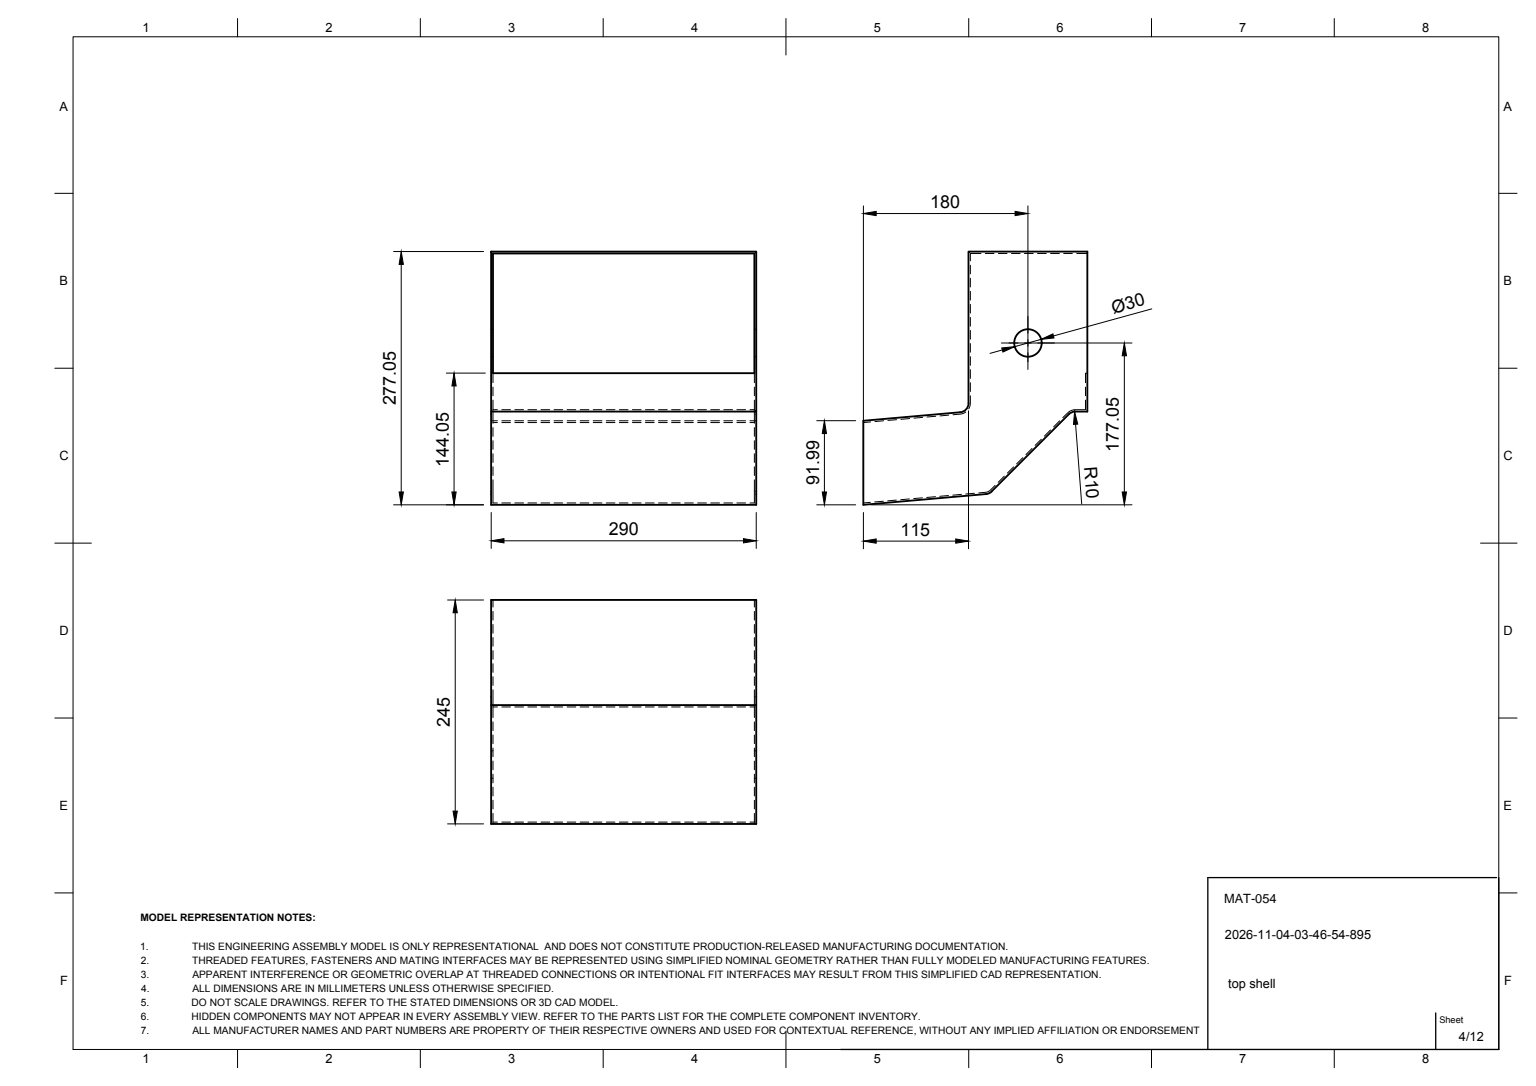
ISO-10303-21;
HEADER;
FILE_DESCRIPTION (('STEP AP214'),
    '1' );
FILE_NAME ('top shell.step',
    '2026-10-21T17:50:41',
    ( '' ),
    ( '' ),
    'SwSTEP 2.0',
    'SolidWorks 2026',
    '' );
FILE_SCHEMA (( 'AUTOMOTIVE_DESIGN' ));
ENDSEC;

DATA;
#13=ORIENTED_EDGE ( 'NONE', *, *, #11369, .F. ) ;
#14=DIRECTION ( 'NONE',  ( 0.000000000000000000, 0.000000000000000000, -1.000000000000000000 ) ) ;
#111=DIRECTION ( 'NONE',  ( -1.000000000000000000, -0.000000000000000000, 0.000000000000000000 ) ) ;
#224=CARTESIAN_POINT ( 'NONE',  ( 143.0000000000000568, -90.29102463692673552, -73.95413108702813076 ) ) ;
#230=LINE ( 'NONE', #27103, #6038 ) ;
#238=DIRECTION ( 'NONE',  ( 0.000000000000000000, 0.000000000000000000, 1.000000000000000000 ) ) ;
#332=VECTOR ( 'NONE', #22185, 999.9999999999998863 ) ;
#381=EDGE_CURVE ( 'NONE', #23842, #27991, #33323, .T. ) ;
#384=CARTESIAN_POINT ( 'NONE',  ( 145.0000000000000568, -87.50000000000000000, 65.00000000000000000 ) ) ;
#404=VERTEX_POINT ( 'NONE', #32954 ) ;
#417=EDGE_CURVE ( 'NONE', #26117, #20828, #25120, .T. ) ;
#450=ORIENTED_EDGE ( 'NONE', *, *, #30527, .F. ) ;
#467=CARTESIAN_POINT ( 'NONE',  ( -145.0000000000000568, -87.50000000000000000, 65.00000000000000000 ) ) ;
#474=VERTEX_POINT ( 'NONE', #30482 ) ;
#477=DIRECTION ( 'NONE',  ( 0.000000000000000000, 0.000000000000000000, 1.000000000000000000 ) ) ;
#478=CARTESIAN_POINT ( 'NONE',  ( 145.0000000000000568, -90.29102463692674974, -73.95413108702814498 ) ) ;
#501=VERTEX_POINT ( 'NONE', #14993 ) ;
#508=EDGE_CURVE ( 'NONE', #6161, #17092, #29208, .T. ) ;
#579=DIRECTION ( 'NONE',  ( -1.000000000000000000, -0.000000000000000000, -0.000000000000000000 ) ) ;
#608=AXIS2_PLACEMENT_3D ( 'NONE', #24658, #22008, #32850 ) ;
#649=FACE_OUTER_BOUND ( 'NONE', #15663, .T. ) ;
#660=VECTOR ( 'NONE', #33698, 1000.000000000000000 ) ;
#691=DIRECTION ( 'NONE',  ( -1.000000000000000000, -0.000000000000000000, -0.000000000000000000 ) ) ;
#694=ORIENTED_EDGE ( 'NONE', *, *, #22904, .F. ) ;
#716=LINE ( 'NONE', #33098, #30982 ) ;
#751=CARTESIAN_POINT ( 'NONE',  ( 143.0000000000000568, -167.8552739801376390, -46.75049602362128809 ) ) ;
#757=DIRECTION ( 'NONE',  ( -1.000000000000000000, -0.000000000000000000, -0.000000000000000000 ) ) ;
#923=ORIENTED_EDGE ( 'NONE', *, *, #10157, .T. ) ;
#932=DIRECTION ( 'NONE',  ( 0.000000000000000000, 0.000000000000000000, -1.000000000000000000 ) ) ;
#975=LINE ( 'NONE', #1321, #16054 ) ;
#984=VERTEX_POINT ( 'NONE', #15788 ) ;
#990=AXIS2_PLACEMENT_3D ( 'NONE', #24668, #10640, #10812 ) ;
#1006=LINE ( 'NONE', #478, #28288 ) ;
#1010=CARTESIAN_POINT ( 'NONE',  ( 145.0000000000000568, -99.56883598056833762, -180.0000000000000000 ) ) ;
#1039=CARTESIAN_POINT ( 'NONE',  ( 187.4264068711928530, -12.50000000000001066, 15.00000000000001243 ) ) ;
#1054=VERTEX_POINT ( 'NONE', #18119 ) ;
#1114=MECHANICAL_DESIGN_GEOMETRIC_PRESENTATION_REPRESENTATION('',(#28951),#30096);
#1116=SHAPE_REPRESENTATION_RELATIONSHIP ( 'NONE' , 'NONE' ,  #34141, #15654 ) ;
#1119=VECTOR ( 'NONE', #9651, 1000.000000000000000 ) ;
#1129=VECTOR ( 'NONE', #24012, 1000.000000000000000 ) ;
#1146=ORIENTED_EDGE ( 'NONE', *, *, #20627, .F. ) ;
#1160=ORIENTED_EDGE ( 'NONE', *, *, #15687, .T. ) ;
#1162=ADVANCED_FACE ( 'NONE', ( #33539, #17379 ), #31058, .F. ) ;
#1184=DIRECTION ( 'NONE',  ( 0.000000000000000000, 0.000000000000000000, 1.000000000000000000 ) ) ;
#1244=ORIENTED_EDGE ( 'NONE', *, *, #5386, .F. ) ;
#1280=DIRECTION ( 'NONE',  ( 0.000000000000000000, 1.000000000000000000, 0.000000000000000000 ) ) ;
#1321=CARTESIAN_POINT ( 'NONE',  ( 145.0000000000000568, -97.56119630548165844, -180.0000000000000000 ) ) ;
#1392=ORIENTED_EDGE ( 'NONE', *, *, #20061, .F. ) ;
#1406=ORIENTED_EDGE ( 'NONE', *, *, #28646, .F. ) ;
#1446=ORIENTED_EDGE ( 'NONE', *, *, #32975, .T. ) ;
#1462=EDGE_CURVE ( 'NONE', #30062, #4232, #230, .T. ) ;
#1493=DIRECTION ( 'NONE',  ( 0.000000000000000000, 0.000000000000000000, 1.000000000000000000 ) ) ;
#1495=EDGE_CURVE ( 'NONE', #13296, #6161, #27458, .T. ) ;
#1497=FACE_OUTER_BOUND ( 'NONE', #34932, .T. ) ;
#1609=ORIENTED_EDGE ( 'NONE', *, *, #17986, .F. ) ;
#1662=CARTESIAN_POINT ( 'NONE',  ( 145.0000000000000568, -167.8552739801376390, -46.75049602362128809 ) ) ;
#1668=CARTESIAN_POINT ( 'NONE',  ( 145.0000000000000568, -97.49999999999998579, 51.88904920397793319 ) ) ;
#1722=VERTEX_POINT ( 'NONE', #2207 ) ;
#1762=ORIENTED_EDGE ( 'NONE', *, *, #9120, .F. ) ;
#1828=VECTOR ( 'NONE', #34629, 1000.000000000000000 ) ;
#1964=ORIENTED_EDGE ( 'NONE', *, *, #8386, .F. ) ;
#1974=DIRECTION ( 'NONE',  ( -1.000000000000000000, -0.000000000000000000, -0.000000000000000000 ) ) ;
#2049=UNCERTAINTY_MEASURE_WITH_UNIT (LENGTH_MEASURE( 1.000000000000000082E-05 ), #3564, 'distance_accuracy_value', 'NONE');
#2074=EDGE_CURVE ( 'NONE', #21429, #4511, #10494, .T. ) ;
#2104=ORIENTED_EDGE ( 'NONE', *, *, #27915, .T. ) ;
#2107=EDGE_LOOP ( 'NONE', ( #4532, #34179, #24526, #34171 ) ) ;
#2147=DIRECTION ( 'NONE',  ( -0.000000000000000000, 1.000000000000000000, 0.000000000000000000 ) ) ;
#2200=DIRECTION ( 'NONE',  ( 0.000000000000000000, 0.000000000000000000, 1.000000000000000000 ) ) ;
#2207=CARTESIAN_POINT ( 'NONE',  ( 143.0000000000000568, -175.8248315648716016, -46.05325008164005851 ) ) ;
#2212=DIRECTION ( 'NONE',  ( 0.000000000000000000, -0.000000000000000000, -1.000000000000000000 ) ) ;
#2216=LINE ( 'NONE', #23916, #17432 ) ;
#2264=ORIENTED_EDGE ( 'NONE', *, *, #32975, .F. ) ;
#2305=FACE_OUTER_BOUND ( 'NONE', #6168, .T. ) ;
#2345=FACE_OUTER_BOUND ( 'NONE', #21509, .T. ) ;
#2382=ORIENTED_EDGE ( 'NONE', *, *, #15611, .F. ) ;
#2386=EDGE_CURVE ( 'NONE', #32063, #28687, #25581, .T. ) ;
#2423=DIRECTION ( 'NONE',  ( 1.000000000000000000, 0.000000000000000000, 0.000000000000000000 ) ) ;
#2439=VERTEX_POINT ( 'NONE', #30935 ) ;
#2538=VECTOR ( 'NONE', #8049, 999.9999999999998863 ) ;
#2546=DIRECTION ( 'NONE',  ( -1.000000000000000000, -0.000000000000000000, -0.000000000000000000 ) ) ;
#2625=DIRECTION ( 'NONE',  ( 0.000000000000000000, 0.000000000000000000, -1.000000000000000000 ) ) ;
#2626=ORIENTED_EDGE ( 'NONE', *, *, #4967, .F. ) ;
#2671=CARTESIAN_POINT ( 'NONE',  ( 145.0000000000000568, -87.50000000000000000, 65.00000000000000000 ) ) ;
#2701=DIRECTION ( 'NONE',  ( 0.000000000000000000, 0.08715574274765885976, 0.9961946980917454342 ) ) ;
#2717=CARTESIAN_POINT ( 'NONE',  ( 145.0000000000000568, -177.8172209610550851, -45.87893859614474223 ) ) ;
#2748=DIRECTION ( 'NONE',  ( -1.000000000000000000, -0.000000000000000000, -0.000000000000000000 ) ) ;
#2766=ADVANCED_FACE ( 'NONE', ( #12390 ), #33735, .T. ) ;
#2827=ORIENTED_EDGE ( 'NONE', *, *, #11782, .F. ) ;
#2895=EDGE_LOOP ( 'NONE', ( #29008, #11211, #28715, #34782, #8518, #32872, #13532, #19129, #17560, #923, #20347, #17292, #33269 ) ) ;
#2907=ADVANCED_FACE ( 'NONE', ( #26592 ), #20740, .T. ) ;
#2992=ORIENTED_EDGE ( 'NONE', *, *, #10272, .F. ) ;
#3001=VERTEX_POINT ( 'NONE', #32627 ) ;
#3070=VECTOR ( 'NONE', #20545, 999.9999999999998863 ) ;
#3081=EDGE_CURVE ( 'NONE', #20828, #6161, #16397, .T. ) ;
#3110=AXIS2_PLACEMENT_3D ( 'NONE', #24223, #10182, #23528 ) ;
#3175=VERTEX_POINT ( 'NONE', #17168 ) ;
#3206=ORIENTED_EDGE ( 'NONE', *, *, #4973, .T. ) ;
#3237=FACE_OUTER_BOUND ( 'NONE', #2895, .T. ) ;
#3262=DIRECTION ( 'NONE',  ( 0.000000000000000000, 0.000000000000000000, -1.000000000000000000 ) ) ;
#3299=DIRECTION ( 'NONE',  ( 0.000000000000000000, 0.000000000000000000, -1.000000000000000000 ) ) ;
#3328=LINE ( 'NONE', #22377, #8717 ) ;
#3329=EDGE_LOOP ( 'NONE', ( #28799, #16866, #1609, #5261 ) ) ;
#3333=ORIENTED_EDGE ( 'NONE', *, *, #18846, .F. ) ;
#3359=EDGE_CURVE ( 'NONE', #26117, #13296, #26604, .T. ) ;
#3458=ORIENTED_EDGE ( 'NONE', *, *, #1462, .F. ) ;
#3475=AXIS2_PLACEMENT_3D ( 'NONE', #25994, #12657, #33480 ) ;
#3486=DIRECTION ( 'NONE',  ( 0.000000000000000000, 0.000000000000000000, -1.000000000000000000 ) ) ;
#3544=CARTESIAN_POINT ( 'NONE',  ( 143.0000000000000568, -78.33668825982573480, -63.00000000000000000 ) ) ;
#3564=( LENGTH_UNIT ( ) NAMED_UNIT ( * ) SI_UNIT ( .MILLI., .METRE. ) );
#3617=DIRECTION ( 'NONE',  ( 0.000000000000000000, -0.7071067811865489050, -0.7071067811865462405 ) ) ;
#3629=CARTESIAN_POINT ( 'NONE',  ( -143.0000000000000568, -12.50000000000001066, 15.00000000000001243 ) ) ;
#3804=LINE ( 'NONE', #31730, #14481 ) ;
#3827=ORIENTED_EDGE ( 'NONE', *, *, #20467, .T. ) ;
#3841=ORIENTED_EDGE ( 'NONE', *, *, #34221, .F. ) ;
#3928=CARTESIAN_POINT ( 'NONE',  ( -143.0000000000000568, -97.49999999999998579, 51.88904920397793319 ) ) ;
#3993=EDGE_CURVE ( 'NONE', #32063, #26390, #6167, .T. ) ;
#3997=VERTEX_POINT ( 'NONE', #33215 ) ;
#4033=FACE_OUTER_BOUND ( 'NONE', #29172, .T. ) ;
#4066=ORIENTED_EDGE ( 'NONE', *, *, #21663, .F. ) ;
#4184=DIRECTION ( 'NONE',  ( -1.000000000000000000, 0.000000000000000000, 0.000000000000000000 ) ) ;
#4232=VERTEX_POINT ( 'NONE', #31760 ) ;
#4285=VECTOR ( 'NONE', #28507, 1000.000000000000227 ) ;
#4334=VECTOR ( 'NONE', #24783, 1000.000000000000000 ) ;
#4350=DIRECTION ( 'NONE',  ( -1.000000000000000000, -0.000000000000000000, -0.000000000000000000 ) ) ;
#4401=LINE ( 'NONE', #15293, #20876 ) ;
#4418=EDGE_LOOP ( 'NONE', ( #13811, #31599, #10235, #6638 ) ) ;
#4435=ORIENTED_EDGE ( 'NONE', *, *, #20467, .F. ) ;
#4440=CARTESIAN_POINT ( 'NONE',  ( -145.0000000000000568, -87.50000000000000000, 65.00000000000000000 ) ) ;
#4461=AXIS2_PLACEMENT_3D ( 'NONE', #31281, #6881, #28959 ) ;
#4511=VERTEX_POINT ( 'NONE', #30683 ) ;
#4532=ORIENTED_EDGE ( 'NONE', *, *, #9727, .F. ) ;
#4600=CIRCLE ( 'NONE', #19406, 12.00000000000001066 ) ;
#4612=VECTOR ( 'NONE', #17082, 1000.000000000000000 ) ;
#4619=DIRECTION ( 'NONE',  ( -1.000000000000000000, -0.000000000000000000, -0.000000000000000000 ) ) ;
#4630=VECTOR ( 'NONE', #18717, 1000.000000000000000 ) ;
#4755=LINE ( 'NONE', #23647, #20022 ) ;
#4847=CARTESIAN_POINT ( 'NONE',  ( -145.0000000000000568, -90.42893218813456713, 44.81798139211241505 ) ) ;
#4920=CARTESIAN_POINT ( 'NONE',  ( 143.0000000000000568, -97.49999999999998579, 51.88904920397793319 ) ) ;
#4933=VECTOR ( 'NONE', #16029, 1000.000000000000000 ) ;
#4967=EDGE_CURVE ( 'NONE', #7013, #474, #20146, .T. ) ;
#4973=EDGE_CURVE ( 'NONE', #17236, #13268, #34177, .T. ) ;
#4975=ORIENTED_EDGE ( 'NONE', *, *, #30527, .T. ) ;
#5002=EDGE_CURVE ( 'NONE', #22371, #14920, #15688, .T. ) ;
#5063=VECTOR ( 'NONE', #28015, 1000.000000000000000 ) ;
#5079=EDGE_CURVE ( 'NONE', #25727, #3001, #15866, .T. ) ;
#5084=ORIENTED_EDGE ( 'NONE', *, *, #1462, .T. ) ;
#5093=ORIENTED_EDGE ( 'NONE', *, *, #27195, .F. ) ;
#5105=LINE ( 'NONE', #15467, #11496 ) ;
#5139=ORIENTED_EDGE ( 'NONE', *, *, #18904, .T. ) ;
#5230=CARTESIAN_POINT ( 'NONE',  ( 187.4264068711928530, -12.50000000000001066, 15.00000000000001243 ) ) ;
#5242=( GEOMETRIC_REPRESENTATION_CONTEXT ( 3 ) GLOBAL_UNCERTAINTY_ASSIGNED_CONTEXT ( ( #9608 ) ) GLOBAL_UNIT_ASSIGNED_CONTEXT ( ( #24956, #11279, #14303 ) ) REPRESENTATION_CONTEXT ( 'NONE', 'WORKASPACE' ) );
#5261=ORIENTED_EDGE ( 'NONE', *, *, #30865, .T. ) ;
#5265=CYLINDRICAL_SURFACE ( 'NONE', #8945, 15.00000000000000000 ) ;
#5298=AXIS2_PLACEMENT_3D ( 'NONE', #3928, #11973, #932 ) ;
#5302=DIRECTION ( 'NONE',  ( 0.000000000000000000, -1.000000000000000000, 0.000000000000000000 ) ) ;
#5362=PLANE ( 'NONE',  #11451 ) ;
#5370=DIRECTION ( 'NONE',  ( 0.000000000000000000, -0.08715574274765887364, -0.9961946980917455452 ) ) ;
#5386=EDGE_CURVE ( 'NONE', #27028, #21429, #20894, .T. ) ;
#5473=ORIENTED_EDGE ( 'NONE', *, *, #17425, .T. ) ;
#5527=ORIENTED_EDGE ( 'NONE', *, *, #22904, .T. ) ;
#5532=CARTESIAN_POINT ( 'NONE',  ( 145.0000000000000568, -78.33668825982573480, -65.00000000000000000 ) ) ;
#5554=EDGE_CURVE ( 'NONE', #474, #20668, #12228, .T. ) ;
#5688=AXIS2_PLACEMENT_3D ( 'NONE', #25048, #691, #6543 ) ;
#5698=ORIENTED_EDGE ( 'NONE', *, *, #27195, .T. ) ;
#5708=CARTESIAN_POINT ( 'NONE',  ( 145.0000000000000568, -90.42893218813456713, 44.81798139211241505 ) ) ;
#5768=PRODUCT ( 'top shell', 'top shell', '', ( #13906 ) ) ;
#5808=PLANE ( 'NONE',  #32666 ) ;
#5937=DIRECTION ( 'NONE',  ( 0.000000000000000000, 0.000000000000000000, -1.000000000000000000 ) ) ;
#5975=DIRECTION ( 'NONE',  ( 1.000000000000000000, 0.000000000000000000, 0.000000000000000000 ) ) ;
#6038=VECTOR ( 'NONE', #29775, 1000.000000000000000 ) ;
#6096=VECTOR ( 'NONE', #5370, 999.9999999999998863 ) ;
#6120=ORIENTED_EDGE ( 'NONE', *, *, #1495, .T. ) ;
#6146=DIRECTION ( 'NONE',  ( -1.000000000000000000, -0.000000000000000000, -0.000000000000000000 ) ) ;
#6161=VERTEX_POINT ( 'NONE', #34700 ) ;
#6167=CIRCLE ( 'NONE', #26071, 15.00000000000000000 ) ;
#6168=EDGE_LOOP ( 'NONE', ( #10986, #30418, #14003, #26658 ) ) ;
#6171=CARTESIAN_POINT ( 'NONE',  ( 145.0000000000000568, 87.50000000000000000, 65.00000000000000000 ) ) ;
#6176=CARTESIAN_POINT ( 'NONE',  ( 187.4264068711928530, -12.50000000000001066, 1.224646799147353217E-14 ) ) ;
#6230=CARTESIAN_POINT ( 'NONE',  ( 145.0000000000000568, -12.50000000000000888, -14.99999999999998757 ) ) ;
#6319=DIRECTION ( 'NONE',  ( 0.000000000000000000, 0.000000000000000000, -1.000000000000000000 ) ) ;
#6352=ORIENTED_EDGE ( 'NONE', *, *, #11580, .F. ) ;
#6420=VECTOR ( 'NONE', #16754, 1000.000000000000000 ) ;
#6429=DIRECTION ( 'NONE',  ( 0.000000000000000000, 0.000000000000000000, 1.000000000000000000 ) ) ;
#6433=DIRECTION ( 'NONE',  ( 0.000000000000000000, 0.000000000000000000, 1.000000000000000000 ) ) ;
#6489=ORIENTED_EDGE ( 'NONE', *, *, #25794, .T. ) ;
#6543=DIRECTION ( 'NONE',  ( 0.000000000000000000, 0.000000000000000000, 1.000000000000000000 ) ) ;
#6555=EDGE_CURVE ( 'NONE', #34864, #26182, #18491, .T. ) ;
#6638=ORIENTED_EDGE ( 'NONE', *, *, #11580, .T. ) ;
#6666=APPLICATION_CONTEXT ( 'automotive_design' ) ;
#6689=DIRECTION ( 'NONE',  ( -1.000000000000000000, -0.000000000000000000, -0.000000000000000000 ) ) ;
#6719=ORIENTED_EDGE ( 'NONE', *, *, #13733, .T. ) ;
#6743=DIRECTION ( 'NONE',  ( 0.000000000000000000, 0.000000000000000000, -1.000000000000000000 ) ) ;
#6829=DIRECTION ( 'NONE',  ( 0.000000000000000000, 0.000000000000000000, -1.000000000000000000 ) ) ;
#6881=DIRECTION ( 'NONE',  ( 1.000000000000000000, 0.000000000000000000, 0.000000000000000000 ) ) ;
#6888=PLANE ( 'NONE',  #26569 ) ;
#6897=EDGE_CURVE ( 'NONE', #14920, #18737, #9189, .T. ) ;
#6925=AXIS2_PLACEMENT_3D ( 'NONE', #13977, #13617, #21623 ) ;
#6945=LINE ( 'NONE', #28674, #14077 ) ;
#6961=EDGE_LOOP ( 'NONE', ( #6719, #4435, #33462, #26506 ) ) ;
#7013=VERTEX_POINT ( 'NONE', #29103 ) ;
#7060=DIRECTION ( 'NONE',  ( 0.000000000000000000, -1.000000000000000000, -3.017235169886638201E-16 ) ) ;
#7152=EDGE_CURVE ( 'NONE', #20668, #9976, #14555, .T. ) ;
#7158=AXIS2_PLACEMENT_3D ( 'NONE', #29451, #28917, #2212 ) ;
#7160=EDGE_LOOP ( 'NONE', ( #34385, #13685 ) ) ;
#7165=CYLINDRICAL_SURFACE ( 'NONE', #27539, 11.99999999999998934 ) ;
#7329=CARTESIAN_POINT ( 'NONE',  ( 145.0000000000000568, -85.49999999999998579, 65.00000000000000000 ) ) ;
#7336=EDGE_CURVE ( 'NONE', #1054, #28789, #25689, .T. ) ;
#7426=DIRECTION ( 'NONE',  ( -1.000000000000000000, 0.000000000000000000, -0.000000000000000000 ) ) ;
#7428=DIRECTION ( 'NONE',  ( -1.000000000000000000, 0.000000000000000000, 0.000000000000000000 ) ) ;
#7533=EDGE_CURVE ( 'NONE', #28789, #25461, #26207, .T. ) ;
#7576=DIRECTION ( 'NONE',  ( 0.000000000000000000, 0.000000000000000000, 1.000000000000000000 ) ) ;
#7600=DIRECTION ( 'NONE',  ( -0.000000000000000000, -0.000000000000000000, 1.000000000000000000 ) ) ;
#7631=ORIENTED_EDGE ( 'NONE', *, *, #16410, .T. ) ;
#7653=DIRECTION ( 'NONE',  ( -1.000000000000000000, -0.000000000000000000, 0.000000000000000000 ) ) ;
#7661=VECTOR ( 'NONE', #7653, 1000.000000000000000 ) ;
#7744=ADVANCED_FACE ( 'NONE', ( #12617 ), #34315, .F. ) ;
#7796=ORIENTED_EDGE ( 'NONE', *, *, #6555, .F. ) ;
#7799=CARTESIAN_POINT ( 'NONE',  ( -145.0000000000000568, -97.56119630548165844, -180.0000000000000000 ) ) ;
#7831=CARTESIAN_POINT ( 'NONE',  ( 187.4264068711928530, -12.50000000000000888, -14.99999999999998757 ) ) ;
#7853=CARTESIAN_POINT ( 'NONE',  ( 145.0000000000000568, -78.33668825982579165, -65.00000000000000000 ) ) ;
#7897=ORIENTED_EDGE ( 'NONE', *, *, #26520, .F. ) ;
#7998=ORIENTED_EDGE ( 'NONE', *, *, #5079, .F. ) ;
#8017=CARTESIAN_POINT ( 'NONE',  ( 145.0000000000000568, -12.50000000000001066, 1.224646799147353217E-14 ) ) ;
#8032=ORIENTED_EDGE ( 'NONE', *, *, #3993, .F. ) ;
#8049=DIRECTION ( 'NONE',  ( 0.000000000000000000, -0.7071067811865489050, -0.7071067811865462405 ) ) ;
#8154=DIRECTION ( 'NONE',  ( -0.000000000000000000, 1.000000000000000000, 3.017235169886638201E-16 ) ) ;
#8183=CARTESIAN_POINT ( 'NONE',  ( 145.0000000000000568, -174.9263417920030577, -39.67942821175577706 ) ) ;
#8223=ADVANCED_FACE ( 'NONE', ( #10750 ), #21599, .F. ) ;
#8236=ORIENTED_EDGE ( 'NONE', *, *, #3081, .F. ) ;
#8265=ADVANCED_FACE ( 'NONE', ( #14903 ), #25558, .F. ) ;
#8280=ORIENTED_EDGE ( 'NONE', *, *, #28479, .F. ) ;
#8304=FACE_OUTER_BOUND ( 'NONE', #24607, .T. ) ;
#8354=ORIENTED_EDGE ( 'NONE', *, *, #10623, .T. ) ;
#8382=EDGE_CURVE ( 'NONE', #18126, #20668, #34989, .T. ) ;
#8386=EDGE_CURVE ( 'NONE', #21429, #26117, #29633, .T. ) ;
#8398=FACE_OUTER_BOUND ( 'NONE', #14678, .T. ) ;
#8425=EDGE_LOOP ( 'NONE', ( #26192, #31699, #27048, #3458, #22844, #27025, #12510, #10788, #3333, #20172, #32420, #23199, #2626 ) ) ;
#8518=ORIENTED_EDGE ( 'NONE', *, *, #26675, .T. ) ;
#8565=PRODUCT_DEFINITION_CONTEXT ( 'detailed design', #6666, 'design' ) ;
#8583=EDGE_CURVE ( 'NONE', #3175, #19641, #21348, .T. ) ;
#8603=LINE ( 'NONE', #19483, #26490 ) ;
#8608=DIRECTION ( 'NONE',  ( 0.000000000000000000, -2.312964634635743450E-15, -1.000000000000000000 ) ) ;
#8717=VECTOR ( 'NONE', #14206, 1000.000000000000000 ) ;
#8727=LINE ( 'NONE', #384, #32402 ) ;
#8773=CARTESIAN_POINT ( 'NONE',  ( 145.0000000000000568, -88.29863524074325198, -74.12844257252345415 ) ) ;
#8799=LINE ( 'NONE', #5230, #17823 ) ;
#8839=AXIS2_PLACEMENT_3D ( 'NONE', #25160, #30692, #5937 ) ;
#8862=AXIS2_PLACEMENT_3D ( 'NONE', #18961, #27482, #8608 ) ;
#8869=ORIENTED_EDGE ( 'NONE', *, *, #2386, .F. ) ;
#8893=DIRECTION ( 'NONE',  ( 0.000000000000000000, 1.000000000000000000, 0.000000000000000000 ) ) ;
#8922=DIRECTION ( 'NONE',  ( 1.000000000000000000, 0.000000000000000000, -0.000000000000000000 ) ) ;
#8928=EDGE_CURVE ( 'NONE', #19525, #25531, #16614, .T. ) ;
#8938=VECTOR ( 'NONE', #5975, 1000.000000000000000 ) ;
#8945=AXIS2_PLACEMENT_3D ( 'NONE', #13829, #13478, #24313 ) ;
#8968=EDGE_CURVE ( 'NONE', #28789, #1722, #26563, .T. ) ;
#9033=DIRECTION ( 'NONE',  ( -0.000000000000000000, -0.000000000000000000, 1.000000000000000000 ) ) ;
#9091=( NAMED_UNIT ( * ) SI_UNIT ( $, .STERADIAN. ) SOLID_ANGLE_UNIT ( ) );
#9110=CARTESIAN_POINT ( 'NONE',  ( -143.0000000000000568, -78.33668825982573480, -63.00000000000000000 ) ) ;
#9120=EDGE_CURVE ( 'NONE', #34290, #10259, #6945, .T. ) ;
#9131=ORIENTED_EDGE ( 'NONE', *, *, #7533, .T. ) ;
#9142=DIRECTION ( 'NONE',  ( 0.000000000000000000, -1.000000000000000000, 0.000000000000000000 ) ) ;
#9189=LINE ( 'NONE', #1010, #19655 ) ;
#9291=CARTESIAN_POINT ( 'NONE',  ( 145.0000000000000568, -174.9263417920030577, -39.67942821175577706 ) ) ;
#9322=CARTESIAN_POINT ( 'NONE',  ( -145.0000000000000568, -174.9263417920030577, -39.67942821175577706 ) ) ;
#9461=DIRECTION ( 'NONE',  ( 0.000000000000000000, 0.000000000000000000, -1.000000000000000000 ) ) ;
#9480=ORIENTED_EDGE ( 'NONE', *, *, #14642, .T. ) ;
#9606=ADVANCED_FACE ( 'NONE', ( #649 ), #16869, .F. ) ;
#9608=UNCERTAINTY_MEASURE_WITH_UNIT (LENGTH_MEASURE( 1.000000000000000082E-05 ), #24956, 'distance_accuracy_value', 'NONE');
#9651=DIRECTION ( 'NONE',  ( 0.000000000000000000, 0.000000000000000000, -1.000000000000000000 ) ) ;
#9702=CARTESIAN_POINT ( 'NONE',  ( 145.0000000000000568, -85.49999999999998579, 51.88904920397798293 ) ) ;
#9727=EDGE_CURVE ( 'NONE', #25531, #18737, #33111, .T. ) ;
#9927=DIRECTION ( 'NONE',  ( 0.000000000000000000, -0.9961946980917453232, 0.08715574274766170471 ) ) ;
#9976=VERTEX_POINT ( 'NONE', #26325 ) ;
#9996=ORIENTED_EDGE ( 'NONE', *, *, #28646, .T. ) ;
#10016=ADVANCED_FACE ( 'NONE', ( #16194 ), #10672, .F. ) ;
#10039=CARTESIAN_POINT ( 'NONE',  ( 145.0000000000000568, -177.8172209610550851, -45.87893859614474223 ) ) ;
#10091=DIRECTION ( 'NONE',  ( -1.000000000000000000, -0.000000000000000000, -0.000000000000000000 ) ) ;
#10152=DIRECTION ( 'NONE',  ( -1.000000000000000000, -0.000000000000000000, -0.000000000000000000 ) ) ;
#10157=EDGE_CURVE ( 'NONE', #3997, #23842, #32882, .T. ) ;
#10182=DIRECTION ( 'NONE',  ( -1.000000000000000000, 0.000000000000000000, 0.000000000000000000 ) ) ;
#10187=DIRECTION ( 'NONE',  ( 1.000000000000000000, 0.000000000000000000, 0.000000000000000000 ) ) ;
#10235=ORIENTED_EDGE ( 'NONE', *, *, #33095, .T. ) ;
#10242=ADVANCED_FACE ( 'NONE', ( #17609, #23110 ), #33954, .F. ) ;
#10259=VERTEX_POINT ( 'NONE', #15446 ) ;
#10272=EDGE_CURVE ( 'NONE', #18752, #27262, #24923, .T. ) ;
#10320=CARTESIAN_POINT ( 'NONE',  ( -145.0000000000000568, -12.50000000000001066, 1.224646799147353217E-14 ) ) ;
#10351=LINE ( 'NONE', #7853, #21315 ) ;
#10369=DIRECTION ( 'NONE',  ( -1.000000000000000000, -0.000000000000000000, -0.000000000000000000 ) ) ;
#10435=ORIENTED_EDGE ( 'NONE', *, *, #7336, .T. ) ;
#10437=AXIS2_PLACEMENT_3D ( 'NONE', #6176, #10091, #33952 ) ;
#10440=ORIENTED_EDGE ( 'NONE', *, *, #20627, .T. ) ;
#10447=AXIS2_PLACEMENT_3D ( 'NONE', #1668, #31901, #34770 ) ;
#10459=CARTESIAN_POINT ( 'NONE',  ( 145.0000000000000568, -87.50000000000000000, 65.00000000000000000 ) ) ;
#10472=PLANE ( 'NONE',  #12121 ) ;
#10494=LINE ( 'NONE', #24180, #28668 ) ;
#10555=CARTESIAN_POINT ( 'NONE',  ( 145.0000000000000568, -78.33668825982573480, -63.00000000000000000 ) ) ;
#10572=EDGE_CURVE ( 'NONE', #10822, #10259, #22718, .T. ) ;
#10623=EDGE_CURVE ( 'NONE', #404, #3001, #12869, .T. ) ;
#10640=DIRECTION ( 'NONE',  ( 0.000000000000000000, -0.9961946980917453232, 0.08715574274766170471 ) ) ;
#10672=PLANE ( 'NONE',  #31709 ) ;
#10750=FACE_OUTER_BOUND ( 'NONE', #17032, .T. ) ;
#10771=ORIENTED_EDGE ( 'NONE', *, *, #33429, .T. ) ;
#10781=VERTEX_POINT ( 'NONE', #21733 ) ;
#10788=ORIENTED_EDGE ( 'NONE', *, *, #5002, .F. ) ;
#10807=CARTESIAN_POINT ( 'NONE',  ( 145.0000000000000568, 85.49999999999998579, -63.00000000000000000 ) ) ;
#10812=DIRECTION ( 'NONE',  ( 0.000000000000000000, -0.08715574274766170471, -0.9961946980917453232 ) ) ;
#10822=VERTEX_POINT ( 'NONE', #21569 ) ;
#10823=MANIFOLD_SOLID_BREP ( 'Cut-Extrude1', #11122 ) ;
#10827=VECTOR ( 'NONE', #17484, 1000.000000000000000 ) ;
#10924=VERTEX_POINT ( 'NONE', #31832 ) ;
#10933=ORIENTED_EDGE ( 'NONE', *, *, #19299, .T. ) ;
#10986=ORIENTED_EDGE ( 'NONE', *, *, #3081, .T. ) ;
#11013=CARTESIAN_POINT ( 'NONE',  ( 0.000000000000000000, -45.49999999999999289, 0.000000000000000000 ) ) ;
#11079=DIRECTION ( 'NONE',  ( 1.000000000000000000, 0.000000000000000000, -0.000000000000000000 ) ) ;
#11122=CLOSED_SHELL ( 'NONE', ( #11469, #8223, #1162, #25891, #31386, #10242, #29405, #13232, #33340, #32574, #20577, #30934, #7744, #11329, #8265, #32213, #29610, #16701, #2907, #20856, #32836, #14670, #9606, #16742, #20637, #2766, #33187, #10016, #14324, #17218 ) ) ;
#11169=CARTESIAN_POINT ( 'NONE',  ( 145.0000000000000568, -90.42893218813456713, 44.81798139211241505 ) ) ;
#11211=ORIENTED_EDGE ( 'NONE', *, *, #31750, .T. ) ;
#11267=AXIS2_PLACEMENT_3D ( 'NONE', #26950, #23918, #13265 ) ;
#11279=( NAMED_UNIT ( * ) PLANE_ANGLE_UNIT ( ) SI_UNIT ( $, .RADIAN. ) );
#11288=CARTESIAN_POINT ( 'NONE',  ( -145.0000000000000568, -167.8552739801376390, -46.75049602362128809 ) ) ;
#11329=ADVANCED_FACE ( 'NONE', ( #34306 ), #6888, .F. ) ;
#11345=LINE ( 'NONE', #16517, #8938 ) ;
#11369=EDGE_CURVE ( 'NONE', #30062, #27991, #21131, .T. ) ;
#11427=ORIENTED_EDGE ( 'NONE', *, *, #8583, .T. ) ;
#11451=AXIS2_PLACEMENT_3D ( 'NONE', #27261, #32069, #2701 ) ;
#11462=DIRECTION ( 'NONE',  ( -1.000000000000000000, -0.000000000000000000, -0.000000000000000000 ) ) ;
#11467=CARTESIAN_POINT ( 'NONE',  ( 145.0000000000000568, -187.5436536988701732, -180.0000000000000284 ) ) ;
#11469=ADVANCED_FACE ( 'NONE', ( #8304 ), #5265, .F. ) ;
#11496=VECTOR ( 'NONE', #7600, 1000.000000000000000 ) ;
#11555=VECTOR ( 'NONE', #19111, 1000.000000000000000 ) ;
#11580=EDGE_CURVE ( 'NONE', #10924, #3997, #1006, .T. ) ;
#11599=( NAMED_UNIT ( * ) PLANE_ANGLE_UNIT ( ) SI_UNIT ( $, .RADIAN. ) );
#11693=DIRECTION ( 'NONE',  ( -1.000000000000000000, -0.000000000000000000, -0.000000000000000000 ) ) ;
#11707=DIRECTION ( 'NONE',  ( 0.000000000000000000, -1.000000000000000000, 0.000000000000000000 ) ) ;
#11756=VECTOR ( 'NONE', #23770, 1000.000000000000000 ) ;
#11782=EDGE_CURVE ( 'NONE', #2439, #4511, #31157, .T. ) ;
#11794=CARTESIAN_POINT ( 'NONE',  ( 145.0000000000000568, -177.8172209610550851, -45.87893859614474223 ) ) ;
#11838=LINE ( 'NONE', #11467, #660 ) ;
#11842=FACE_OUTER_BOUND ( 'NONE', #15543, .T. ) ;
#11871=DIRECTION ( 'NONE',  ( -1.000000000000000000, -0.000000000000000000, -0.000000000000000000 ) ) ;
#11875=LINE ( 'NONE', #30367, #332 ) ;
#11908=DIRECTION ( 'NONE',  ( -1.000000000000000000, -0.000000000000000000, -0.000000000000000000 ) ) ;
#11973=DIRECTION ( 'NONE',  ( 1.000000000000000000, 0.000000000000000000, 0.000000000000000000 ) ) ;
#12121=AXIS2_PLACEMENT_3D ( 'NONE', #34499, #2625, #7426 ) ;
#12179=EDGE_LOOP ( 'NONE', ( #24309, #27182, #1244, #3827 ) ) ;
#12228=LINE ( 'NONE', #9702, #34536 ) ;
#12247=VECTOR ( 'NONE', #23635, 1000.000000000000000 ) ;
#12254=ORIENTED_EDGE ( 'NONE', *, *, #26324, .T. ) ;
#12330=CARTESIAN_POINT ( 'NONE',  ( 143.0000000000000568, -12.50000000000000888, -14.99999999999998757 ) ) ;
#12334=EDGE_LOOP ( 'NONE', ( #15230, #13, #5084, #32622 ) ) ;
#12379=CARTESIAN_POINT ( 'NONE',  ( 145.0000000000000568, -97.56119630548165844, -180.0000000000000000 ) ) ;
#12390=FACE_OUTER_BOUND ( 'NONE', #12960, .T. ) ;
#12496=VECTOR ( 'NONE', #13183, 999.9999999999998863 ) ;
#12510=ORIENTED_EDGE ( 'NONE', *, *, #33095, .F. ) ;
#12617=FACE_OUTER_BOUND ( 'NONE', #25678, .T. ) ;
#12656=DIRECTION ( 'NONE',  ( -0.000000000000000000, 1.000000000000000000, 3.017235169886638201E-16 ) ) ;
#12657=DIRECTION ( 'NONE',  ( 1.000000000000000000, 0.000000000000000000, 0.000000000000000000 ) ) ;
#12696=VERTEX_POINT ( 'NONE', #14376 ) ;
#12719=PLANE ( 'NONE',  #10447 ) ;
#12794=DIRECTION ( 'NONE',  ( -1.000000000000000000, -0.000000000000000000, -0.000000000000000000 ) ) ;
#12808=EDGE_LOOP ( 'NONE', ( #1146, #32235, #28832, #22275 ) ) ;
#12826=VECTOR ( 'NONE', #9033, 1000.000000000000000 ) ;
#12869=LINE ( 'NONE', #13042, #24369 ) ;
#12929=CARTESIAN_POINT ( 'NONE',  ( -143.0000000000000568, -85.49999999999998579, 65.00000000000000000 ) ) ;
#12934=ORIENTED_EDGE ( 'NONE', *, *, #15611, .T. ) ;
#12960=EDGE_LOOP ( 'NONE', ( #24836, #6352, #23231, #10771 ) ) ;
#12995=DIRECTION ( 'NONE',  ( -1.000000000000000000, -0.000000000000000000, -0.000000000000000000 ) ) ;
#13009=CARTESIAN_POINT ( 'NONE',  ( -143.0000000000000568, -45.49999999999999289, 51.88904920397793319 ) ) ;
#13027=CARTESIAN_POINT ( 'NONE',  ( 187.4264068711928530, -12.50000000000000888, -14.99999999999998757 ) ) ;
#13042=CARTESIAN_POINT ( 'NONE',  ( 145.0000000000000568, -88.29863524074325198, -74.12844257252345415 ) ) ;
#13073=DIRECTION ( 'NONE',  ( 1.000000000000000000, 0.000000000000000000, 0.000000000000000000 ) ) ;
#13131=EDGE_CURVE ( 'NONE', #4232, #501, #14690, .T. ) ;
#13183=DIRECTION ( 'NONE',  ( -0.000000000000000000, 0.08715574274766170471, 0.9961946980917453232 ) ) ;
#13203=AXIS2_PLACEMENT_3D ( 'NONE', #1662, #34715, #1493 ) ;
#13232=ADVANCED_FACE ( 'NONE', ( #11842 ), #22691, .F. ) ;
#13255=ORIENTED_EDGE ( 'NONE', *, *, #5554, .T. ) ;
#13265=DIRECTION ( 'NONE',  ( 0.000000000000000000, 0.000000000000000000, -1.000000000000000000 ) ) ;
#13268=VERTEX_POINT ( 'NONE', #25691 ) ;
#13296=VERTEX_POINT ( 'NONE', #31045 ) ;
#13360=LINE ( 'NONE', #13009, #4933 ) ;
#13459=VECTOR ( 'NONE', #10152, 1000.000000000000000 ) ;
#13470=DIRECTION ( 'NONE',  ( 0.000000000000000000, 0.000000000000000000, -1.000000000000000000 ) ) ;
#13478=DIRECTION ( 'NONE',  ( -1.000000000000000000, -0.000000000000000000, -0.000000000000000000 ) ) ;
#13532=ORIENTED_EDGE ( 'NONE', *, *, #8928, .T. ) ;
#13556=VECTOR ( 'NONE', #12656, 1000.000000000000000 ) ;
#13579=DIRECTION ( 'NONE',  ( 1.000000000000000000, 0.000000000000000000, 0.000000000000000000 ) ) ;
#13588=ORIENTED_EDGE ( 'NONE', *, *, #13733, .F. ) ;
#13617=DIRECTION ( 'NONE',  ( 1.000000000000000000, 0.000000000000000000, 0.000000000000000000 ) ) ;
#13685=ORIENTED_EDGE ( 'NONE', *, *, #30624, .T. ) ;
#13719=DIRECTION ( 'NONE',  ( -1.000000000000000000, -0.000000000000000000, -0.000000000000000000 ) ) ;
#13721=EDGE_LOOP ( 'NONE', ( #694, #27702, #25001, #28605 ) ) ;
#13733=EDGE_CURVE ( 'NONE', #13268, #2439, #23348, .T. ) ;
#13797=CARTESIAN_POINT ( 'NONE',  ( -143.0000000000000568, -173.5121282296299796, -41.09364177412887642 ) ) ;
#13811=ORIENTED_EDGE ( 'NONE', *, *, #19213, .F. ) ;
#13819=DIRECTION ( 'NONE',  ( 0.000000000000000000, 1.000000000000000000, 0.000000000000000000 ) ) ;
#13823=FACE_OUTER_BOUND ( 'NONE', #15394, .T. ) ;
#13829=CARTESIAN_POINT ( 'NONE',  ( 187.4264068711928530, -12.50000000000001066, 1.224646799147353217E-14 ) ) ;
#13834=DIRECTION ( 'NONE',  ( 0.000000000000000000, 0.7071067811865489050, 0.7071067811865462405 ) ) ;
#13906=PRODUCT_CONTEXT ( 'NONE', #18084, 'mechanical' ) ;
#13915=ORIENTED_EDGE ( 'NONE', *, *, #21663, .T. ) ;
#13947=EDGE_CURVE ( 'NONE', #26182, #13268, #8727, .T. ) ;
#13960=ORIENTED_EDGE ( 'NONE', *, *, #24814, .F. ) ;
#13977=CARTESIAN_POINT ( 'NONE',  ( 143.0000000000000568, -12.50000000000001066, 1.224646799147353217E-14 ) ) ;
#14003=ORIENTED_EDGE ( 'NONE', *, *, #3359, .F. ) ;
#14077=VECTOR ( 'NONE', #17141, 1000.000000000000000 ) ;
#14084=EDGE_CURVE ( 'NONE', #501, #10781, #17817, .T. ) ;
#14100=FACE_OUTER_BOUND ( 'NONE', #21791, .T. ) ;
#14159=AXIS2_PLACEMENT_3D ( 'NONE', #33595, #27902, #19561 ) ;
#14176=CARTESIAN_POINT ( 'NONE',  ( 145.0000000000000568, -97.49999999999998579, 51.88904920397793319 ) ) ;
#14206=DIRECTION ( 'NONE',  ( -0.000000000000000000, 0.000000000000000000, 1.000000000000000000 ) ) ;
#14261=CIRCLE ( 'NONE', #26177, 15.00000000000000000 ) ;
#14300=CARTESIAN_POINT ( 'NONE',  ( -145.0000000000000568, -78.33668825982579165, -75.00000000000001421 ) ) ;
#14303=( NAMED_UNIT ( * ) SI_UNIT ( $, .STERADIAN. ) SOLID_ANGLE_UNIT ( ) );
#14324=ADVANCED_FACE ( 'NONE', ( #4033 ), #30936, .F. ) ;
#14376=CARTESIAN_POINT ( 'NONE',  ( 145.0000000000000568, -189.5512933739568666, -180.0000000000000284 ) ) ;
#14394=CARTESIAN_POINT ( 'NONE',  ( -143.0000000000000568, 85.49999999999998579, -63.00000000000000000 ) ) ;
#14437=LINE ( 'NONE', #19418, #6420 ) ;
#14441=ORIENTED_EDGE ( 'NONE', *, *, #34524, .T. ) ;
#14476=DIRECTION ( 'NONE',  ( -1.000000000000000000, -0.000000000000000000, 0.000000000000000000 ) ) ;
#14481=VECTOR ( 'NONE', #31392, 1000.000000000000000 ) ;
#14555=CIRCLE ( 'NONE', #8862, 11.99999999999999645 ) ;
#14564=VECTOR ( 'NONE', #579, 1000.000000000000000 ) ;
#14639=FACE_BOUND ( 'NONE', #19295, .T. ) ;
#14642=EDGE_CURVE ( 'NONE', #26390, #32063, #14261, .T. ) ;
#14670=ADVANCED_FACE ( 'NONE', ( #13823 ), #21482, .T. ) ;
#14678=EDGE_LOOP ( 'NONE', ( #21999, #450, #20457, #7631 ) ) ;
#14690=LINE ( 'NONE', #30689, #5063 ) ;
#14819=PLANE ( 'NONE',  #20166 ) ;
#14874=ORIENTED_EDGE ( 'NONE', *, *, #5386, .T. ) ;
#14876=AXIS2_PLACEMENT_3D ( 'NONE', #10555, #26733, #11079 ) ;
#14903=FACE_OUTER_BOUND ( 'NONE', #22837, .T. ) ;
#14920=VERTEX_POINT ( 'NONE', #34438 ) ;
#14955=CARTESIAN_POINT ( 'NONE',  ( 143.0000000000000568, -78.33668825982579165, -63.00000000000000000 ) ) ;
#14992=CARTESIAN_POINT ( 'NONE',  ( -144.4704739938196099, -45.49999999999999289, 63.00000000000000000 ) ) ;
#14993=CARTESIAN_POINT ( 'NONE',  ( 143.0000000000000568, -45.49999999999999289, 65.00000000000000000 ) ) ;
#15010=ORIENTED_EDGE ( 'NONE', *, *, #30694, .T. ) ;
#15155=PLANE ( 'NONE',  #3475 ) ;
#15169=CARTESIAN_POINT ( 'NONE',  ( 143.0000000000000568, -78.33668825982579165, -75.00000000000001421 ) ) ;
#15196=ORIENTED_EDGE ( 'NONE', *, *, #8382, .F. ) ;
#15230=ORIENTED_EDGE ( 'NONE', *, *, #31529, .F. ) ;
#15293=CARTESIAN_POINT ( 'NONE',  ( 145.0000000000000568, -87.50000000000000000, 51.88904920397797582 ) ) ;
#15302=CARTESIAN_POINT ( 'NONE',  ( -143.0000000000000568, -12.50000000000000888, -14.99999999999998757 ) ) ;
#15309=ORIENTED_EDGE ( 'NONE', *, *, #19299, .F. ) ;
#15320=ORIENTED_EDGE ( 'NONE', *, *, #508, .T. ) ;
#15327=DIRECTION ( 'NONE',  ( -1.000000000000000000, 0.000000000000000000, 0.000000000000000000 ) ) ;
#15394=EDGE_LOOP ( 'NONE', ( #19316, #2382, #10435, #9131 ) ) ;
#15415=ORIENTED_EDGE ( 'NONE', *, *, #24814, .T. ) ;
#15446=CARTESIAN_POINT ( 'NONE',  ( -145.0000000000000568, 87.50000000000000000, -65.00000000000000000 ) ) ;
#15467=CARTESIAN_POINT ( 'NONE',  ( -145.0000000000000568, 87.50000000000000000, 65.00000000000000000 ) ) ;
#15503=LINE ( 'NONE', #26519, #13459 ) ;
#15543=EDGE_LOOP ( 'NONE', ( #15415, #29772, #20086, #17085 ) ) ;
#15565=VECTOR ( 'NONE', #8893, 1000.000000000000000 ) ;
#15578=ORIENTED_EDGE ( 'NONE', *, *, #18287, .T. ) ;
#15590=AXIS2_PLACEMENT_3D ( 'NONE', #28340, #757, #6429 ) ;
#15611=EDGE_CURVE ( 'NONE', #1054, #9976, #33962, .T. ) ;
#15654=ADVANCED_BREP_SHAPE_REPRESENTATION ( '', ( #10823, #28566 ), #5242 ) ;
#15663=EDGE_LOOP ( 'NONE', ( #7897, #24334, #17855, #4975 ) ) ;
#15687=EDGE_CURVE ( 'NONE', #474, #1054, #34134, .T. ) ;
#15688=LINE ( 'NONE', #28669, #13556 ) ;
#15703=LINE ( 'NONE', #13027, #28666 ) ;
#15731=EDGE_LOOP ( 'NONE', ( #19928, #3841, #7998, #25452, #29923, #8236, #2264, #2827, #13588, #34164, #13960 ) ) ;
#15788=CARTESIAN_POINT ( 'NONE',  ( 145.0000000000000568, -97.56119630548165844, -180.0000000000000000 ) ) ;
#15798=VECTOR ( 'NONE', #32500, 1000.000000000000000 ) ;
#15814=CARTESIAN_POINT ( 'NONE',  ( 143.0000000000000568, -12.50000000000001066, 15.00000000000001243 ) ) ;
#15866=LINE ( 'NONE', #20832, #12496 ) ;
#16029=DIRECTION ( 'NONE',  ( 0.000000000000000000, 0.000000000000000000, -1.000000000000000000 ) ) ;
#16054=VECTOR ( 'NONE', #17188, 1000.000000000000000 ) ;
#16126=LINE ( 'NONE', #27134, #23430 ) ;
#16194=FACE_OUTER_BOUND ( 'NONE', #25084, .T. ) ;
#16214=VECTOR ( 'NONE', #11908, 1000.000000000000000 ) ;
#16241=ORIENTED_EDGE ( 'NONE', *, *, #17986, .T. ) ;
#16344=FACE_OUTER_BOUND ( 'NONE', #19275, .T. ) ;
#16397=CIRCLE ( 'NONE', #28320, 9.999999999999994671 ) ;
#16410=EDGE_CURVE ( 'NONE', #22371, #25531, #11838, .T. ) ;
#16511=CARTESIAN_POINT ( 'NONE',  ( -143.0000000000000568, -99.56883598056833762, -180.0000000000000000 ) ) ;
#16517=CARTESIAN_POINT ( 'NONE',  ( -144.4704739938196099, -45.49999999999999289, 65.00000000000000000 ) ) ;
#16523=ORIENTED_EDGE ( 'NONE', *, *, #29246, .F. ) ;
#16527=DIRECTION ( 'NONE',  ( 0.000000000000000000, -0.000000000000000000, 1.000000000000000000 ) ) ;
#16614=LINE ( 'NONE', #33319, #6096 ) ;
#16616=CARTESIAN_POINT ( 'NONE',  ( 143.0000000000000568, -97.49999999999998579, 63.00000000000000000 ) ) ;
#16634=DIRECTION ( 'NONE',  ( -0.000000000000000000, 0.08715574274766170471, 0.9961946980917453232 ) ) ;
#16701=ADVANCED_FACE ( 'NONE', ( #2345 ), #21405, .T. ) ;
#16704=FACE_OUTER_BOUND ( 'NONE', #6961, .T. ) ;
#16730=CIRCLE ( 'NONE', #22406, 10.00000000000000888 ) ;
#16742=ADVANCED_FACE ( 'NONE', ( #8398 ), #5362, .T. ) ;
#16754=DIRECTION ( 'NONE',  ( -1.000000000000000000, -0.000000000000000000, -0.000000000000000000 ) ) ;
#16783=PLANE ( 'NONE',  #31865 ) ;
#16788=CIRCLE ( 'NONE', #3110, 15.00000000000000000 ) ;
#16814=ORIENTED_EDGE ( 'NONE', *, *, #16963, .T. ) ;
#16823=DIRECTION ( 'NONE',  ( 1.000000000000000000, 0.000000000000000000, 0.000000000000000000 ) ) ;
#16866=ORIENTED_EDGE ( 'NONE', *, *, #10623, .F. ) ;
#16869=CYLINDRICAL_SURFACE ( 'NONE', #21516, 7.999999999999992895 ) ;
#16963=EDGE_CURVE ( 'NONE', #17092, #25727, #21681, .T. ) ;
#16981=CARTESIAN_POINT ( 'NONE',  ( 145.0000000000000568, -87.50000000000000000, 51.88904920397797582 ) ) ;
#16997=ORIENTED_EDGE ( 'NONE', *, *, #3993, .T. ) ;
#17032=EDGE_LOOP ( 'NONE', ( #16997, #5698, #26447, #8869 ) ) ;
#17064=ORIENTED_EDGE ( 'NONE', *, *, #14084, .T. ) ;
#17082=DIRECTION ( 'NONE',  ( -1.000000000000000000, 0.000000000000000000, -0.000000000000000000 ) ) ;
#17085=ORIENTED_EDGE ( 'NONE', *, *, #9120, .T. ) ;
#17092=VERTEX_POINT ( 'NONE', #19559 ) ;
#17103=AXIS2_PLACEMENT_3D ( 'NONE', #8017, #13719, #14 ) ;
#17135=ORIENTED_EDGE ( 'NONE', *, *, #30865, .F. ) ;
#17141=DIRECTION ( 'NONE',  ( -1.000000000000000000, -0.000000000000000000, -0.000000000000000000 ) ) ;
#17145=DIRECTION ( 'NONE',  ( -0.000000000000000000, 0.08715574274766170471, 0.9961946980917453232 ) ) ;
#17168=CARTESIAN_POINT ( 'NONE',  ( 145.0000000000000568, -12.50000000000001066, 15.00000000000001243 ) ) ;
#17188=DIRECTION ( 'NONE',  ( -1.000000000000000000, -0.000000000000000000, -0.000000000000000000 ) ) ;
#17218=ADVANCED_FACE ( 'NONE', ( #19732 ), #30585, .F. ) ;
#17236=VERTEX_POINT ( 'NONE', #33778 ) ;
#17292=ORIENTED_EDGE ( 'NONE', *, *, #31529, .T. ) ;
#17301=CARTESIAN_POINT ( 'NONE',  ( 143.0000000000000568, -45.49999999999999289, 51.88904920397793319 ) ) ;
#17379=FACE_OUTER_BOUND ( 'NONE', #8425, .T. ) ;
#17425=EDGE_CURVE ( 'NONE', #404, #26887, #16730, .T. ) ;
#17432=VECTOR ( 'NONE', #34796, 999.9999999999998863 ) ;
#17484=DIRECTION ( 'NONE',  ( 0.000000000000000000, 0.000000000000000000, -1.000000000000000000 ) ) ;
#17510=CYLINDRICAL_SURFACE ( 'NONE', #15590, 9.999999999999994671 ) ;
#17560=ORIENTED_EDGE ( 'NONE', *, *, #19213, .T. ) ;
#17603=VECTOR ( 'NONE', #13819, 1000.000000000000000 ) ;
#17609=FACE_OUTER_BOUND ( 'NONE', #24389, .T. ) ;
#17777=ORIENTED_EDGE ( 'NONE', *, *, #34221, .T. ) ;
#17779=ORIENTED_EDGE ( 'NONE', *, *, #34524, .F. ) ;
#17817=LINE ( 'NONE', #17301, #10827 ) ;
#17823=VECTOR ( 'NONE', #21624, 1000.000000000000000 ) ;
#17855=ORIENTED_EDGE ( 'NONE', *, *, #8968, .T. ) ;
#17860=AXIS2_PLACEMENT_3D ( 'NONE', #28811, #20290, #6743 ) ;
#17961=VECTOR ( 'NONE', #6319, 1000.000000000000000 ) ;
#17986=EDGE_CURVE ( 'NONE', #984, #404, #22491, .T. ) ;
#18032=AXIS2_PLACEMENT_3D ( 'NONE', #10320, #15327, #29547 ) ;
#18080=LINE ( 'NONE', #12379, #20569 ) ;
#18084=APPLICATION_CONTEXT ( 'automotive_design' ) ;
#18119=CARTESIAN_POINT ( 'NONE',  ( 143.0000000000000568, -89.01471862576147487, 43.40376782973931569 ) ) ;
#18126=VERTEX_POINT ( 'NONE', #31027 ) ;
#18224=DIRECTION ( 'NONE',  ( -0.000000000000000000, 1.000000000000000000, 0.000000000000000000 ) ) ;
#18287=EDGE_CURVE ( 'NONE', #28687, #22784, #16788, .T. ) ;
#18346=EDGE_CURVE ( 'NONE', #26887, #10822, #10351, .T. ) ;
#18491=LINE ( 'NONE', #10459, #12247 ) ;
#18520=VECTOR ( 'NONE', #32466, 999.9999999999998863 ) ;
#18575=CARTESIAN_POINT ( 'NONE',  ( -143.0000000000000568, -175.8248315648716016, -46.05325008164005851 ) ) ;
#18717=DIRECTION ( 'NONE',  ( -1.000000000000000000, -0.000000000000000000, -0.000000000000000000 ) ) ;
#18737=VERTEX_POINT ( 'NONE', #16511 ) ;
#18738=DIRECTION ( 'NONE',  ( -1.000000000000000000, -0.000000000000000000, -0.000000000000000000 ) ) ;
#18752=VERTEX_POINT ( 'NONE', #15814 ) ;
#18846=EDGE_CURVE ( 'NONE', #1722, #22371, #11875, .T. ) ;
#18904=EDGE_CURVE ( 'NONE', #26182, #27028, #22362, .T. ) ;
#18961=CARTESIAN_POINT ( 'NONE',  ( -143.0000000000000568, -97.49999999999998579, 51.88904920397793319 ) ) ;
#18993=PRODUCT_DEFINITION_FORMATION_WITH_SPECIFIED_SOURCE ( 'ANY', '', #5768, .NOT_KNOWN. ) ;
#19100=DIRECTION ( 'NONE',  ( 0.000000000000000000, 0.000000000000000000, 1.000000000000000000 ) ) ;
#19107=VECTOR ( 'NONE', #1280, 1000.000000000000000 ) ;
#19111=DIRECTION ( 'NONE',  ( 0.000000000000000000, -1.000000000000000000, 0.000000000000000000 ) ) ;
#19118=CARTESIAN_POINT ( 'NONE',  ( -143.0000000000000568, 85.49999999999998579, 65.00000000000000000 ) ) ;
#19129=ORIENTED_EDGE ( 'NONE', *, *, #9727, .T. ) ;
#19213=EDGE_CURVE ( 'NONE', #18737, #3997, #2216, .T. ) ;
#19255=VECTOR ( 'NONE', #9461, 1000.000000000000000 ) ;
#19275=EDGE_LOOP ( 'NONE', ( #1446, #21063, #1964, #34424 ) ) ;
#19295=EDGE_LOOP ( 'NONE', ( #19501, #1392 ) ) ;
#19299=EDGE_CURVE ( 'NONE', #7013, #18126, #8603, .T. ) ;
#19316=ORIENTED_EDGE ( 'NONE', *, *, #26675, .F. ) ;
#19406=AXIS2_PLACEMENT_3D ( 'NONE', #15169, #1974, #32040 ) ;
#19411=LINE ( 'NONE', #3544, #15565 ) ;
#19418=CARTESIAN_POINT ( 'NONE',  ( -144.4704739938196099, -45.49999999999999289, 63.00000000000000000 ) ) ;
#19454=LINE ( 'NONE', #16616, #11555 ) ;
#19483=CARTESIAN_POINT ( 'NONE',  ( -144.4704739938196099, -85.49999999999998579, 63.00000000000000000 ) ) ;
#19501=ORIENTED_EDGE ( 'NONE', *, *, #18287, .F. ) ;
#19525=VERTEX_POINT ( 'NONE', #18575 ) ;
#19559=CARTESIAN_POINT ( 'NONE',  ( -145.0000000000000568, -189.5512933739568666, -180.0000000000000284 ) ) ;
#19561=DIRECTION ( 'NONE',  ( 0.000000000000000000, 2.312964634635740689E-15, -1.000000000000000000 ) ) ;
#19641=VERTEX_POINT ( 'NONE', #6230 ) ;
#19655=VECTOR ( 'NONE', #4184, 1000.000000000000000 ) ;
#19732=FACE_OUTER_BOUND ( 'NONE', #13721, .T. ) ;
#19928=ORIENTED_EDGE ( 'NONE', *, *, #10572, .F. ) ;
#19979=FACE_OUTER_BOUND ( 'NONE', #12179, .T. ) ;
#20022=VECTOR ( 'NONE', #7428, 1000.000000000000000 ) ;
#20045=ORIENTED_EDGE ( 'NONE', *, *, #7152, .F. ) ;
#20053=ORIENTED_EDGE ( 'NONE', *, *, #5554, .F. ) ;
#20061=EDGE_CURVE ( 'NONE', #22784, #28687, #31102, .T. ) ;
#20071=EDGE_CURVE ( 'NONE', #23024, #27819, #13360, .T. ) ;
#20086=ORIENTED_EDGE ( 'NONE', *, *, #27915, .F. ) ;
#20089=VECTOR ( 'NONE', #11707, 1000.000000000000000 ) ;
#20146=LINE ( 'NONE', #30991, #19255 ) ;
#20161=ORIENTED_EDGE ( 'NONE', *, *, #4967, .T. ) ;
#20166=AXIS2_PLACEMENT_3D ( 'NONE', #14992, #28506, #26169 ) ;
#20172=ORIENTED_EDGE ( 'NONE', *, *, #8968, .F. ) ;
#20267=CARTESIAN_POINT ( 'NONE',  ( 145.0000000000000568, -97.56119630548165844, -180.0000000000000000 ) ) ;
#20290=DIRECTION ( 'NONE',  ( 1.000000000000000000, 0.000000000000000000, 0.000000000000000000 ) ) ;
#20347=ORIENTED_EDGE ( 'NONE', *, *, #381, .T. ) ;
#20372=CARTESIAN_POINT ( 'NONE',  ( -143.0000000000000568, -187.5436536988702017, -180.0000000000000284 ) ) ;
#20379=LINE ( 'NONE', #22701, #3070 ) ;
#20381=CARTESIAN_POINT ( 'NONE',  ( 143.0000000000000568, -97.49999999999998579, 51.88904920397793319 ) ) ;
#20457=ORIENTED_EDGE ( 'NONE', *, *, #18846, .T. ) ;
#20467=EDGE_CURVE ( 'NONE', #27028, #2439, #4401, .T. ) ;
#20545=DIRECTION ( 'NONE',  ( 0.000000000000000000, -0.7071067811865489050, -0.7071067811865462405 ) ) ;
#20569=VECTOR ( 'NONE', #23227, 1000.000000000000000 ) ;
#20577=ADVANCED_FACE ( 'NONE', ( #16344 ), #22192, .F. ) ;
#20627=EDGE_CURVE ( 'NONE', #23024, #501, #11345, .T. ) ;
#20637=ADVANCED_FACE ( 'NONE', ( #30194 ), #21495, .T. ) ;
#20668=VERTEX_POINT ( 'NONE', #29854 ) ;
#20740=PLANE ( 'NONE',  #7158 ) ;
#20828=VERTEX_POINT ( 'NONE', #9322 ) ;
#20832=CARTESIAN_POINT ( 'NONE',  ( -145.0000000000000568, -88.29863524074325198, -74.12844257252345415 ) ) ;
#20856=ADVANCED_FACE ( 'NONE', ( #31043 ), #31723, .T. ) ;
#20876=VECTOR ( 'NONE', #12794, 1000.000000000000000 ) ;
#20894=CIRCLE ( 'NONE', #23167, 9.999999999999994671 ) ;
#21037=DIRECTION ( 'NONE',  ( 0.000000000000000000, 0.000000000000000000, -1.000000000000000000 ) ) ;
#21055=LINE ( 'NONE', #4847, #2538 ) ;
#21063=ORIENTED_EDGE ( 'NONE', *, *, #417, .F. ) ;
#21131=LINE ( 'NONE', #10807, #15798 ) ;
#21164=DIRECTION ( 'NONE',  ( 0.000000000000000000, -0.000000000000000000, -1.000000000000000000 ) ) ;
#21194=AXIS2_PLACEMENT_3D ( 'NONE', #14300, #14476, #6433 ) ;
#21215=CARTESIAN_POINT ( 'NONE',  ( 145.0000000000000568, -167.8552739801376390, -46.75049602362128809 ) ) ;
#21315=VECTOR ( 'NONE', #18738, 1000.000000000000000 ) ;
#21348=CIRCLE ( 'NONE', #8839, 15.00000000000000000 ) ;
#21373=VECTOR ( 'NONE', #10369, 1000.000000000000000 ) ;
#21405=PLANE ( 'NONE',  #14876 ) ;
#21429=VERTEX_POINT ( 'NONE', #5708 ) ;
#21482=PLANE ( 'NONE',  #608 ) ;
#21495=PLANE ( 'NONE',  #990 ) ;
#21509=EDGE_LOOP ( 'NONE', ( #34616, #28966, #12254, #29796 ) ) ;
#21516=AXIS2_PLACEMENT_3D ( 'NONE', #30020, #11693, #477 ) ;
#21569=CARTESIAN_POINT ( 'NONE',  ( -145.0000000000000568, -78.33668825982579165, -65.00000000000000000 ) ) ;
#21599=CYLINDRICAL_SURFACE ( 'NONE', #30257, 15.00000000000000000 ) ;
#21623=DIRECTION ( 'NONE',  ( 0.000000000000000000, 0.000000000000000000, -1.000000000000000000 ) ) ;
#21624=DIRECTION ( 'NONE',  ( -1.000000000000000000, -0.000000000000000000, -0.000000000000000000 ) ) ;
#21663=EDGE_CURVE ( 'NONE', #12696, #17092, #15503, .T. ) ;
#21681=LINE ( 'NONE', #7799, #32018 ) ;
#21711=CYLINDRICAL_SURFACE ( 'NONE', #13203, 9.999999999999994671 ) ;
#21733=CARTESIAN_POINT ( 'NONE',  ( 143.0000000000000568, -45.49999999999999289, 63.00000000000000000 ) ) ;
#21791=EDGE_LOOP ( 'NONE', ( #23127, #1762, #23558, #31120 ) ) ;
#21937=LINE ( 'NONE', #224, #30394 ) ;
#21999=ORIENTED_EDGE ( 'NONE', *, *, #8928, .F. ) ;
#22008=DIRECTION ( 'NONE',  ( 0.000000000000000000, 0.7071067811865462405, -0.7071067811865489050 ) ) ;
#22089=DIRECTION ( 'NONE',  ( -1.000000000000000000, -0.000000000000000000, -0.000000000000000000 ) ) ;
#22117=EDGE_CURVE ( 'NONE', #3175, #18752, #8799, .T. ) ;
#22174=DIRECTION ( 'NONE',  ( -1.000000000000000000, -0.000000000000000000, -0.000000000000000000 ) ) ;
#22185=DIRECTION ( 'NONE',  ( 0.000000000000000000, -0.08715574274765887364, -0.9961946980917455452 ) ) ;
#22192=PLANE ( 'NONE',  #33373 ) ;
#22275=ORIENTED_EDGE ( 'NONE', *, *, #13131, .T. ) ;
#22362=LINE ( 'NONE', #30552, #17961 ) ;
#22365=DIRECTION ( 'NONE',  ( 1.000000000000000000, 0.000000000000000000, 0.000000000000000000 ) ) ;
#22371=VERTEX_POINT ( 'NONE', #28889 ) ;
#22377=CARTESIAN_POINT ( 'NONE',  ( -143.0000000000000568, 85.49999999999998579, 65.00000000000000000 ) ) ;
#22406=AXIS2_PLACEMENT_3D ( 'NONE', #24469, #111, #7576 ) ;
#22491=LINE ( 'NONE', #8773, #25266 ) ;
#22680=ORIENTED_EDGE ( 'NONE', *, *, #31750, .F. ) ;
#22691=PLANE ( 'NONE',  #32356 ) ;
#22701=CARTESIAN_POINT ( 'NONE',  ( -143.0000000000000568, -89.01471862576147487, 43.40376782973931569 ) ) ;
#22718=LINE ( 'NONE', #33554, #17603 ) ;
#22784=VERTEX_POINT ( 'NONE', #26877 ) ;
#22837=EDGE_LOOP ( 'NONE', ( #17777, #29699, #26457, #8354 ) ) ;
#22844=ORIENTED_EDGE ( 'NONE', *, *, #26324, .F. ) ;
#22904=EDGE_CURVE ( 'NONE', #19641, #27262, #32220, .T. ) ;
#22952=PRODUCT_DEFINITION ( 'UNKNOWN', '', #18993, #8565 ) ;
#23024=VERTEX_POINT ( 'NONE', #27582 ) ;
#23045=CARTESIAN_POINT ( 'NONE',  ( 145.0000000000000568, -97.49999999999998579, 51.88904920397793319 ) ) ;
#23110=FACE_BOUND ( 'NONE', #2107, .T. ) ;
#23121=EDGE_CURVE ( 'NONE', #4232, #26941, #4755, .T. ) ;
#23127=ORIENTED_EDGE ( 'NONE', *, *, #10572, .T. ) ;
#23167=AXIS2_PLACEMENT_3D ( 'NONE', #14176, #22174, #3299 ) ;
#23199=ORIENTED_EDGE ( 'NONE', *, *, #15687, .F. ) ;
#23216=DIRECTION ( 'NONE',  ( -1.000000000000000000, -0.000000000000000000, -0.000000000000000000 ) ) ;
#23227=DIRECTION ( 'NONE',  ( -0.000000000000000000, 1.000000000000000000, 3.017235169886638201E-16 ) ) ;
#23231=ORIENTED_EDGE ( 'NONE', *, *, #23714, .T. ) ;
#23348=LINE ( 'NONE', #467, #1119 ) ;
#23430=VECTOR ( 'NONE', #2748, 1000.000000000000000 ) ;
#23493=ORIENTED_EDGE ( 'NONE', *, *, #14642, .F. ) ;
#23507=FACE_OUTER_BOUND ( 'NONE', #28790, .T. ) ;
#23528=DIRECTION ( 'NONE',  ( 0.000000000000000000, 0.000000000000000000, 1.000000000000000000 ) ) ;
#23558=ORIENTED_EDGE ( 'NONE', *, *, #27521, .F. ) ;
#23635=DIRECTION ( 'NONE',  ( -0.000000000000000000, -1.000000000000000000, -0.000000000000000000 ) ) ;
#23640=DIRECTION ( 'NONE',  ( 0.000000000000000000, 0.9961946980917455452, -0.08715574274765887364 ) ) ;
#23647=CARTESIAN_POINT ( 'NONE',  ( 145.0000000000000568, 85.49999999999998579, 65.00000000000000000 ) ) ;
#23714=EDGE_CURVE ( 'NONE', #10924, #27638, #4600, .T. ) ;
#23770=DIRECTION ( 'NONE',  ( 0.000000000000000000, 0.000000000000000000, -1.000000000000000000 ) ) ;
#23776=VECTOR ( 'NONE', #25622, 1000.000000000000000 ) ;
#23805=CARTESIAN_POINT ( 'NONE',  ( 145.0000000000000568, -88.29863524074325198, -74.12844257252345415 ) ) ;
#23842=VERTEX_POINT ( 'NONE', #24908 ) ;
#23886=CARTESIAN_POINT ( 'NONE',  ( 145.0000000000000568, -173.5121282296299796, -41.09364177412887642 ) ) ;
#23916=CARTESIAN_POINT ( 'NONE',  ( -143.0000000000000568, -90.29102463692673552, -73.95413108702813076 ) ) ;
#23918=DIRECTION ( 'NONE',  ( -1.000000000000000000, -0.000000000000000000, -0.000000000000000000 ) ) ;
#24012=DIRECTION ( 'NONE',  ( -0.000000000000000000, -1.000000000000000000, -0.000000000000000000 ) ) ;
#24064=CARTESIAN_POINT ( 'NONE',  ( -145.0000000000000568, -97.56119630548165844, -180.0000000000000000 ) ) ;
#24167=ORIENTED_EDGE ( 'NONE', *, *, #28479, .T. ) ;
#24180=CARTESIAN_POINT ( 'NONE',  ( 145.0000000000000568, -90.42893218813456713, 44.81798139211241505 ) ) ;
#24223=CARTESIAN_POINT ( 'NONE',  ( -145.0000000000000568, -12.50000000000001066, 1.224646799147353217E-14 ) ) ;
#24309=ORIENTED_EDGE ( 'NONE', *, *, #11782, .T. ) ;
#24313=DIRECTION ( 'NONE',  ( 0.000000000000000000, 0.000000000000000000, 1.000000000000000000 ) ) ;
#24334=ORIENTED_EDGE ( 'NONE', *, *, #7533, .F. ) ;
#24369=VECTOR ( 'NONE', #31874, 1000.000000000000000 ) ;
#24389=EDGE_LOOP ( 'NONE', ( #16814, #17135, #8280, #13915 ) ) ;
#24447=CARTESIAN_POINT ( 'NONE',  ( 145.0000000000000568, -90.42893218813456713, 44.81798139211241505 ) ) ;
#24469=CARTESIAN_POINT ( 'NONE',  ( 145.0000000000000568, -78.33668825982579165, -75.00000000000001421 ) ) ;
#24526=ORIENTED_EDGE ( 'NONE', *, *, #5002, .T. ) ;
#24597=CARTESIAN_POINT ( 'NONE',  ( 187.4264068711928530, -12.50000000000001066, 1.224646799147353217E-14 ) ) ;
#24607=EDGE_LOOP ( 'NONE', ( #1406, #5527, #2992, #26936 ) ) ;
#24658=CARTESIAN_POINT ( 'NONE',  ( 145.0000000000000568, -89.01471862576147487, 43.40376782973931569 ) ) ;
#24668=CARTESIAN_POINT ( 'NONE',  ( 145.0000000000000568, -90.29102463692673552, -73.95413108702813076 ) ) ;
#24781=CARTESIAN_POINT ( 'NONE',  ( 145.0000000000000568, -78.33668825982579165, -65.00000000000000000 ) ) ;
#24783=DIRECTION ( 'NONE',  ( -1.000000000000000000, -0.000000000000000000, -0.000000000000000000 ) ) ;
#24809=AXIS2_PLACEMENT_3D ( 'NONE', #30909, #6689, #1184 ) ;
#24814=EDGE_CURVE ( 'NONE', #10259, #17236, #5105, .T. ) ;
#24836=ORIENTED_EDGE ( 'NONE', *, *, #10157, .F. ) ;
#24858=AXIS2_PLACEMENT_3D ( 'NONE', #751, #13579, #27267 ) ;
#24873=ORIENTED_EDGE ( 'NONE', *, *, #3359, .T. ) ;
#24908=CARTESIAN_POINT ( 'NONE',  ( -143.0000000000000568, -78.33668825982579165, -63.00000000000000000 ) ) ;
#24923=CIRCLE ( 'NONE', #4461, 15.00000000000000000 ) ;
#24956=( LENGTH_UNIT ( ) NAMED_UNIT ( * ) SI_UNIT ( .MILLI., .METRE. ) );
#25001=ORIENTED_EDGE ( 'NONE', *, *, #22117, .T. ) ;
#25048=CARTESIAN_POINT ( 'NONE',  ( 187.4264068711928530, -12.50000000000001066, 1.224646799147353217E-14 ) ) ;
#25084=EDGE_LOOP ( 'NONE', ( #10440, #17064, #14441, #27299 ) ) ;
#25117=FACE_BOUND ( 'NONE', #26661, .T. ) ;
#25120=LINE ( 'NONE', #9291, #14564 ) ;
#25160=CARTESIAN_POINT ( 'NONE',  ( 145.0000000000000568, -12.50000000000001066, 1.224646799147353217E-14 ) ) ;
#25186=DIRECTION ( 'NONE',  ( 0.000000000000000000, 0.000000000000000000, 1.000000000000000000 ) ) ;
#25208=CARTESIAN_POINT ( 'NONE',  ( -143.0000000000000568, -97.49999999999998579, 63.00000000000000000 ) ) ;
#25266=VECTOR ( 'NONE', #16634, 999.9999999999998863 ) ;
#25301=PLANE ( 'NONE',  #5298 ) ;
#25322=VECTOR ( 'NONE', #3617, 999.9999999999998863 ) ;
#25421=CARTESIAN_POINT ( 'NONE',  ( 143.0000000000000568, -173.5121282296299796, -41.09364177412887642 ) ) ;
#25452=ORIENTED_EDGE ( 'NONE', *, *, #16963, .F. ) ;
#25461=VERTEX_POINT ( 'NONE', #13797 ) ;
#25531=VERTEX_POINT ( 'NONE', #20372 ) ;
#25558=CYLINDRICAL_SURFACE ( 'NONE', #24809, 10.00000000000000888 ) ;
#25581=LINE ( 'NONE', #1039, #16214 ) ;
#25610=CIRCLE ( 'NONE', #17103, 15.00000000000000000 ) ;
#25622=DIRECTION ( 'NONE',  ( -0.000000000000000000, 1.000000000000000000, 3.017235169886638201E-16 ) ) ;
#25678=EDGE_LOOP ( 'NONE', ( #15320, #4066, #16523, #6120 ) ) ;
#25689=LINE ( 'NONE', #28193, #25322 ) ;
#25691=CARTESIAN_POINT ( 'NONE',  ( -145.0000000000000568, -87.50000000000000000, 65.00000000000000000 ) ) ;
#25727=VERTEX_POINT ( 'NONE', #24064 ) ;
#25794=EDGE_CURVE ( 'NONE', #10781, #7013, #19454, .T. ) ;
#25815=CIRCLE ( 'NONE', #17860, 7.999999999999992895 ) ;
#25891=ADVANCED_FACE ( 'NONE', ( #25117, #3237 ), #25301, .T. ) ;
#25994=CARTESIAN_POINT ( 'NONE',  ( -145.0000000000000568, -97.49999999999998579, 51.88904920397793319 ) ) ;
#26030=ORIENTED_EDGE ( 'NONE', *, *, #13947, .F. ) ;
#26071=AXIS2_PLACEMENT_3D ( 'NONE', #32370, #22365, #3486 ) ;
#26117=VERTEX_POINT ( 'NONE', #8183 ) ;
#26169=DIRECTION ( 'NONE',  ( 1.000000000000000000, 0.000000000000000000, -0.000000000000000000 ) ) ;
#26177=AXIS2_PLACEMENT_3D ( 'NONE', #26814, #2423, #13470 ) ;
#26182=VERTEX_POINT ( 'NONE', #2671 ) ;
#26192=ORIENTED_EDGE ( 'NONE', *, *, #25794, .F. ) ;
#26207=LINE ( 'NONE', #23886, #21373 ) ;
#26227=DIRECTION ( 'NONE',  ( 0.000000000000000000, -0.08715574274765885976, -0.9961946980917454342 ) ) ;
#26324=EDGE_CURVE ( 'NONE', #27638, #30062, #19411, .T. ) ;
#26325=CARTESIAN_POINT ( 'NONE',  ( -143.0000000000000568, -89.01471862576147487, 43.40376782973931569 ) ) ;
#26390=VERTEX_POINT ( 'NONE', #15302 ) ;
#26447=ORIENTED_EDGE ( 'NONE', *, *, #20061, .T. ) ;
#26457=ORIENTED_EDGE ( 'NONE', *, *, #17425, .F. ) ;
#26468=DIRECTION ( 'NONE',  ( 0.000000000000000000, -2.312964634635743450E-15, -1.000000000000000000 ) ) ;
#26490=VECTOR ( 'NONE', #11462, 1000.000000000000000 ) ;
#26506=ORIENTED_EDGE ( 'NONE', *, *, #13947, .T. ) ;
#26519=CARTESIAN_POINT ( 'NONE',  ( 145.0000000000000568, -189.5512933739568666, -180.0000000000000284 ) ) ;
#26520=EDGE_CURVE ( 'NONE', #25461, #19525, #25815, .T. ) ;
#26563=CIRCLE ( 'NONE', #24858, 7.999999999999992895 ) ;
#26569=AXIS2_PLACEMENT_3D ( 'NONE', #23805, #9927, #34484 ) ;
#26579=CARTESIAN_POINT ( 'NONE',  ( 0.000000000000000000, 0.000000000000000000, 0.000000000000000000 ) ) ;
#26592=FACE_OUTER_BOUND ( 'NONE', #12334, .T. ) ;
#26604=CIRCLE ( 'NONE', #28862, 9.999999999999994671 ) ;
#26658=ORIENTED_EDGE ( 'NONE', *, *, #417, .T. ) ;
#26660=FACE_OUTER_BOUND ( 'NONE', #26817, .T. ) ;
#26661=EDGE_LOOP ( 'NONE', ( #8032, #23493 ) ) ;
#26675=EDGE_CURVE ( 'NONE', #9976, #25461, #20379, .T. ) ;
#26733=DIRECTION ( 'NONE',  ( 0.000000000000000000, 0.000000000000000000, 1.000000000000000000 ) ) ;
#26814=CARTESIAN_POINT ( 'NONE',  ( -143.0000000000000568, -12.50000000000001066, 1.224646799147353217E-14 ) ) ;
#26817=EDGE_LOOP ( 'NONE', ( #3206, #26030, #7796, #15010 ) ) ;
#26877=CARTESIAN_POINT ( 'NONE',  ( -145.0000000000000568, -12.50000000000000888, -14.99999999999998757 ) ) ;
#26887=VERTEX_POINT ( 'NONE', #24781 ) ;
#26936=ORIENTED_EDGE ( 'NONE', *, *, #22117, .F. ) ;
#26941=VERTEX_POINT ( 'NONE', #19118 ) ;
#26950=CARTESIAN_POINT ( 'NONE',  ( -145.0000000000000568, -97.49999999999998579, 51.88904920397793319 ) ) ;
#27025=ORIENTED_EDGE ( 'NONE', *, *, #23714, .F. ) ;
#27028=VERTEX_POINT ( 'NONE', #16981 ) ;
#27048=ORIENTED_EDGE ( 'NONE', *, *, #13131, .F. ) ;
#27103=CARTESIAN_POINT ( 'NONE',  ( 143.0000000000000568, 85.49999999999998579, 65.00000000000000000 ) ) ;
#27134=CARTESIAN_POINT ( 'NONE',  ( 145.0000000000000568, 87.50000000000000000, 65.00000000000000000 ) ) ;
#27182=ORIENTED_EDGE ( 'NONE', *, *, #2074, .F. ) ;
#27195=EDGE_CURVE ( 'NONE', #26390, #22784, #15703, .T. ) ;
#27261=CARTESIAN_POINT ( 'NONE',  ( 145.0000000000000568, -175.8248315648716016, -46.05325008164006562 ) ) ;
#27262=VERTEX_POINT ( 'NONE', #12330 ) ;
#27267=DIRECTION ( 'NONE',  ( 0.000000000000000000, 0.000000000000000000, -1.000000000000000000 ) ) ;
#27299=ORIENTED_EDGE ( 'NONE', *, *, #20071, .F. ) ;
#27458=LINE ( 'NONE', #2717, #4334 ) ;
#27482=DIRECTION ( 'NONE',  ( -1.000000000000000000, -0.000000000000000000, -0.000000000000000000 ) ) ;
#27521=EDGE_CURVE ( 'NONE', #26887, #34290, #716, .T. ) ;
#27539=AXIS2_PLACEMENT_3D ( 'NONE', #23045, #23216, #31221 ) ;
#27582=CARTESIAN_POINT ( 'NONE',  ( -143.0000000000000568, -45.49999999999999289, 65.00000000000000000 ) ) ;
#27638=VERTEX_POINT ( 'NONE', #14955 ) ;
#27700=DIRECTION ( 'NONE',  ( 0.000000000000000000, 0.7071067811865462405, -0.7071067811865489050 ) ) ;
#27702=ORIENTED_EDGE ( 'NONE', *, *, #8583, .F. ) ;
#27819=VERTEX_POINT ( 'NONE', #35046 ) ;
#27822=EDGE_LOOP ( 'NONE', ( #11427, #9996 ) ) ;
#27902=DIRECTION ( 'NONE',  ( -1.000000000000000000, -0.000000000000000000, -0.000000000000000000 ) ) ;
#27915=EDGE_CURVE ( 'NONE', #34290, #34864, #32879, .T. ) ;
#27991=VERTEX_POINT ( 'NONE', #14394 ) ;
#28015=DIRECTION ( 'NONE',  ( 0.000000000000000000, -1.000000000000000000, 0.000000000000000000 ) ) ;
#28129=CARTESIAN_POINT ( 'NONE',  ( -143.0000000000000568, -97.56119630548165844, -180.0000000000000000 ) ) ;
#28193=CARTESIAN_POINT ( 'NONE',  ( 143.0000000000000568, -89.01471862576147487, 43.40376782973931569 ) ) ;
#28208=AXIS2_PLACEMENT_3D ( 'NONE', #11794, #23640, #30650 ) ;
#28277=AXIS2_PLACEMENT_3D ( 'NONE', #7329, #18224, #29054 ) ;
#28288=VECTOR ( 'NONE', #6146, 1000.000000000000000 ) ;
#28320=AXIS2_PLACEMENT_3D ( 'NONE', #11288, #16823, #3262 ) ;
#28340=CARTESIAN_POINT ( 'NONE',  ( 145.0000000000000568, -97.49999999999998579, 51.88904920397793319 ) ) ;
#28431=LINE ( 'NONE', #10039, #34249 ) ;
#28451=ORIENTED_EDGE ( 'NONE', *, *, #29246, .T. ) ;
#28479=EDGE_CURVE ( 'NONE', #12696, #984, #18080, .T. ) ;
#28506=DIRECTION ( 'NONE',  ( 0.000000000000000000, 0.000000000000000000, 1.000000000000000000 ) ) ;
#28507=DIRECTION ( 'NONE',  ( 0.000000000000000000, -0.08715574274765885976, -0.9961946980917454342 ) ) ;
#28566=AXIS2_PLACEMENT_3D ( 'NONE', #26579, #2200, #13073 ) ;
#28605=ORIENTED_EDGE ( 'NONE', *, *, #30624, .F. ) ;
#28646=EDGE_CURVE ( 'NONE', #19641, #3175, #25610, .T. ) ;
#28666=VECTOR ( 'NONE', #4619, 1000.000000000000000 ) ;
#28668=VECTOR ( 'NONE', #12995, 1000.000000000000000 ) ;
#28669=CARTESIAN_POINT ( 'NONE',  ( 143.0000000000000568, -97.56119630548165844, -180.0000000000000000 ) ) ;
#28674=CARTESIAN_POINT ( 'NONE',  ( 145.0000000000000568, 87.50000000000000000, -65.00000000000000000 ) ) ;
#28687=VERTEX_POINT ( 'NONE', #32752 ) ;
#28715=ORIENTED_EDGE ( 'NONE', *, *, #8382, .T. ) ;
#28789=VERTEX_POINT ( 'NONE', #25421 ) ;
#28790=EDGE_LOOP ( 'NONE', ( #17779, #6489, #10933, #22680 ) ) ;
#28799=ORIENTED_EDGE ( 'NONE', *, *, #5079, .T. ) ;
#28811=CARTESIAN_POINT ( 'NONE',  ( -143.0000000000000568, -167.8552739801376390, -46.75049602362128809 ) ) ;
#28832=ORIENTED_EDGE ( 'NONE', *, *, #23121, .F. ) ;
#28862=AXIS2_PLACEMENT_3D ( 'NONE', #21215, #10187, #21037 ) ;
#28889=CARTESIAN_POINT ( 'NONE',  ( 143.0000000000000568, -187.5436536988702017, -180.0000000000000284 ) ) ;
#28917=DIRECTION ( 'NONE',  ( 0.000000000000000000, -1.000000000000000000, 0.000000000000000000 ) ) ;
#28951=STYLED_ITEM('',(#35268),#10823);
#28959=DIRECTION ( 'NONE',  ( 0.000000000000000000, 0.000000000000000000, -1.000000000000000000 ) ) ;
#28966=ORIENTED_EDGE ( 'NONE', *, *, #33429, .F. ) ;
#29008=ORIENTED_EDGE ( 'NONE', *, *, #20071, .T. ) ;
#29054=DIRECTION ( 'NONE',  ( 0.000000000000000000, -0.000000000000000000, 1.000000000000000000 ) ) ;
#29103=CARTESIAN_POINT ( 'NONE',  ( 143.0000000000000568, -85.49999999999998579, 63.00000000000000000 ) ) ;
#29107=CARTESIAN_POINT ( 'NONE',  ( 145.0000000000000568, -175.8248315648716016, -46.05325008164005851 ) ) ;
#29172=EDGE_LOOP ( 'NONE', ( #5093, #9480, #33449, #15578 ) ) ;
#29208=LINE ( 'NONE', #34366, #4285 ) ;
#29246=EDGE_CURVE ( 'NONE', #13296, #12696, #28431, .T. ) ;
#29384=CARTESIAN_POINT ( 'NONE',  ( 145.0000000000000568, -87.50000000000000000, 65.00000000000000000 ) ) ;
#29405=ADVANCED_FACE ( 'NONE', ( #14100 ), #16783, .F. ) ;
#29451=CARTESIAN_POINT ( 'NONE',  ( 145.0000000000000568, 85.49999999999998579, 65.00000000000000000 ) ) ;
#29547=DIRECTION ( 'NONE',  ( 0.000000000000000000, 0.000000000000000000, 1.000000000000000000 ) ) ;
#29610=ADVANCED_FACE ( 'NONE', ( #14639, #31510 ), #15155, .F. ) ;
#29633=LINE ( 'NONE', #24447, #18520 ) ;
#29699=ORIENTED_EDGE ( 'NONE', *, *, #18346, .F. ) ;
#29772=ORIENTED_EDGE ( 'NONE', *, *, #30694, .F. ) ;
#29775=DIRECTION ( 'NONE',  ( -0.000000000000000000, 0.000000000000000000, 1.000000000000000000 ) ) ;
#29796=ORIENTED_EDGE ( 'NONE', *, *, #11369, .T. ) ;
#29854=CARTESIAN_POINT ( 'NONE',  ( -143.0000000000000568, -85.49999999999998579, 51.88904920397798293 ) ) ;
#29923=ORIENTED_EDGE ( 'NONE', *, *, #508, .F. ) ;
#29939=AXIS2_PLACEMENT_3D ( 'NONE', #20381, #33718, #6829 ) ;
#30020=CARTESIAN_POINT ( 'NONE',  ( 145.0000000000000568, -167.8552739801376390, -46.75049602362128809 ) ) ;
#30062=VERTEX_POINT ( 'NONE', #34495 ) ;
#30096=( GEOMETRIC_REPRESENTATION_CONTEXT ( 3 ) GLOBAL_UNCERTAINTY_ASSIGNED_CONTEXT ( ( #2049 ) ) GLOBAL_UNIT_ASSIGNED_CONTEXT ( ( #3564, #11599, #9091 ) ) REPRESENTATION_CONTEXT ( 'NONE', 'WORKASPACE' ) );
#30194=FACE_OUTER_BOUND ( 'NONE', #4418, .T. ) ;
#30205=LINE ( 'NONE', #32038, #7661 ) ;
#30221=AXIS2_PLACEMENT_3D ( 'NONE', #4920, #32163, #26468 ) ;
#30257=AXIS2_PLACEMENT_3D ( 'NONE', #24597, #2546, #238 ) ;
#30266=ORIENTED_EDGE ( 'NONE', *, *, #27521, .T. ) ;
#30367=CARTESIAN_POINT ( 'NONE',  ( 143.0000000000000568, -175.8248315648716016, -46.05325008164006562 ) ) ;
#30394=VECTOR ( 'NONE', #17145, 999.9999999999998863 ) ;
#30418=ORIENTED_EDGE ( 'NONE', *, *, #1495, .F. ) ;
#30482=CARTESIAN_POINT ( 'NONE',  ( 143.0000000000000568, -85.49999999999998579, 51.88904920397798293 ) ) ;
#30527=EDGE_CURVE ( 'NONE', #1722, #19525, #34098, .T. ) ;
#30552=CARTESIAN_POINT ( 'NONE',  ( 145.0000000000000568, -87.50000000000000000, 65.00000000000000000 ) ) ;
#30575=CARTESIAN_POINT ( 'NONE',  ( 145.0000000000000568, 87.50000000000000000, 65.00000000000000000 ) ) ;
#30585=CYLINDRICAL_SURFACE ( 'NONE', #10437, 15.00000000000000000 ) ;
#30624=EDGE_CURVE ( 'NONE', #27262, #18752, #30829, .T. ) ;
#30650=DIRECTION ( 'NONE',  ( 0.000000000000000000, 0.08715574274765885976, 0.9961946980917454342 ) ) ;
#30683=CARTESIAN_POINT ( 'NONE',  ( -145.0000000000000568, -90.42893218813456713, 44.81798139211241505 ) ) ;
#30689=CARTESIAN_POINT ( 'NONE',  ( 143.0000000000000568, -87.50000000000000000, 65.00000000000000000 ) ) ;
#30692=DIRECTION ( 'NONE',  ( -1.000000000000000000, -0.000000000000000000, -0.000000000000000000 ) ) ;
#30694=EDGE_CURVE ( 'NONE', #34864, #17236, #16126, .T. ) ;
#30719=CARTESIAN_POINT ( 'NONE',  ( 145.0000000000000568, -78.33668825982579165, -75.00000000000001421 ) ) ;
#30829=CIRCLE ( 'NONE', #6925, 15.00000000000000000 ) ;
#30865=EDGE_CURVE ( 'NONE', #984, #25727, #975, .T. ) ;
#30909=CARTESIAN_POINT ( 'NONE',  ( 145.0000000000000568, -78.33668825982579165, -75.00000000000001421 ) ) ;
#30934=ADVANCED_FACE ( 'NONE', ( #2305 ), #21711, .T. ) ;
#30935=CARTESIAN_POINT ( 'NONE',  ( -145.0000000000000568, -87.50000000000000000, 51.88904920397797582 ) ) ;
#30936=CYLINDRICAL_SURFACE ( 'NONE', #5688, 15.00000000000000000 ) ;
#30982=VECTOR ( 'NONE', #33282, 1000.000000000000000 ) ;
#30991=CARTESIAN_POINT ( 'NONE',  ( 143.0000000000000568, -85.49999999999998579, 65.00000000000000000 ) ) ;
#31027=CARTESIAN_POINT ( 'NONE',  ( -143.0000000000000568, -85.49999999999998579, 63.00000000000000000 ) ) ;
#31043=FACE_OUTER_BOUND ( 'NONE', #31358, .T. ) ;
#31045=CARTESIAN_POINT ( 'NONE',  ( 145.0000000000000568, -177.8172209610550851, -45.87893859614474223 ) ) ;
#31058=PLANE ( 'NONE',  #29939 ) ;
#31102=CIRCLE ( 'NONE', #18032, 15.00000000000000000 ) ;
#31120=ORIENTED_EDGE ( 'NONE', *, *, #18346, .T. ) ;
#31157=CIRCLE ( 'NONE', #11267, 9.999999999999994671 ) ;
#31188=CARTESIAN_POINT ( 'NONE',  ( 145.0000000000000568, 87.50000000000000000, -65.00000000000000000 ) ) ;
#31221=DIRECTION ( 'NONE',  ( 0.000000000000000000, 0.000000000000000000, 1.000000000000000000 ) ) ;
#31281=CARTESIAN_POINT ( 'NONE',  ( 143.0000000000000568, -12.50000000000001066, 1.224646799147353217E-14 ) ) ;
#31288=CARTESIAN_POINT ( 'NONE',  ( 145.0000000000000568, -89.01471862576147487, 43.40376782973931569 ) ) ;
#31358=EDGE_LOOP ( 'NONE', ( #15309, #20161, #13255, #15196 ) ) ;
#31386=ADVANCED_FACE ( 'NONE', ( #34863, #26660 ), #10472, .F. ) ;
#31392=DIRECTION ( 'NONE',  ( 0.000000000000000000, -1.000000000000000000, 0.000000000000000000 ) ) ;
#31434=LINE ( 'NONE', #25208, #20089 ) ;
#31510=FACE_OUTER_BOUND ( 'NONE', #15731, .T. ) ;
#31529=EDGE_CURVE ( 'NONE', #27991, #26941, #3328, .T. ) ;
#31599=ORIENTED_EDGE ( 'NONE', *, *, #6897, .F. ) ;
#31699=ORIENTED_EDGE ( 'NONE', *, *, #14084, .F. ) ;
#31709=AXIS2_PLACEMENT_3D ( 'NONE', #11013, #5302, #21164 ) ;
#31723=PLANE ( 'NONE',  #28277 ) ;
#31730=CARTESIAN_POINT ( 'NONE',  ( -143.0000000000000568, -87.50000000000000000, 65.00000000000000000 ) ) ;
#31733=FACE_OUTER_BOUND ( 'NONE', #32807, .T. ) ;
#31737=AXIS2_PLACEMENT_3D ( 'NONE', #20267, #34478, #7060 ) ;
#31750=EDGE_CURVE ( 'NONE', #27819, #18126, #31434, .T. ) ;
#31760=CARTESIAN_POINT ( 'NONE',  ( 143.0000000000000568, 85.49999999999998579, 65.00000000000000000 ) ) ;
#31832=CARTESIAN_POINT ( 'NONE',  ( 143.0000000000000568, -90.29102463692674974, -73.95413108702814498 ) ) ;
#31865=AXIS2_PLACEMENT_3D ( 'NONE', #5532, #19100, #8922 ) ;
#31874=DIRECTION ( 'NONE',  ( -1.000000000000000000, -0.000000000000000000, -0.000000000000000000 ) ) ;
#31901=DIRECTION ( 'NONE',  ( 1.000000000000000000, 0.000000000000000000, 0.000000000000000000 ) ) ;
#32018=VECTOR ( 'NONE', #8154, 1000.000000000000000 ) ;
#32038=CARTESIAN_POINT ( 'NONE',  ( 145.0000000000000568, -78.33668825982579165, -63.00000000000000000 ) ) ;
#32040=DIRECTION ( 'NONE',  ( 0.000000000000000000, 2.312964634635740689E-15, -1.000000000000000000 ) ) ;
#32063=VERTEX_POINT ( 'NONE', #3629 ) ;
#32069=DIRECTION ( 'NONE',  ( 0.000000000000000000, 0.9961946980917455452, -0.08715574274765887364 ) ) ;
#32084=FACE_BOUND ( 'NONE', #27822, .T. ) ;
#32163=DIRECTION ( 'NONE',  ( -1.000000000000000000, -0.000000000000000000, -0.000000000000000000 ) ) ;
#32213=ADVANCED_FACE ( 'NONE', ( #32084, #31733 ), #12719, .T. ) ;
#32220=LINE ( 'NONE', #7831, #4630 ) ;
#32235=ORIENTED_EDGE ( 'NONE', *, *, #32793, .F. ) ;
#32356=AXIS2_PLACEMENT_3D ( 'NONE', #33526, #9142, #32816 ) ;
#32370=CARTESIAN_POINT ( 'NONE',  ( -143.0000000000000568, -12.50000000000001066, 1.224646799147353217E-14 ) ) ;
#32402=VECTOR ( 'NONE', #22089, 1000.000000000000000 ) ;
#32420=ORIENTED_EDGE ( 'NONE', *, *, #7336, .F. ) ;
#32466=DIRECTION ( 'NONE',  ( 0.000000000000000000, -0.7071067811865489050, -0.7071067811865462405 ) ) ;
#32500=DIRECTION ( 'NONE',  ( -1.000000000000000000, 0.000000000000000000, 0.000000000000000000 ) ) ;
#32563=CIRCLE ( 'NONE', #21194, 10.00000000000000888 ) ;
#32574=ADVANCED_FACE ( 'NONE', ( #19979 ), #17510, .F. ) ;
#32622=ORIENTED_EDGE ( 'NONE', *, *, #23121, .T. ) ;
#32627=CARTESIAN_POINT ( 'NONE',  ( -145.0000000000000568, -88.29863524074325198, -74.12844257252345415 ) ) ;
#32666=AXIS2_PLACEMENT_3D ( 'NONE', #29384, #2147, #16527 ) ;
#32752=CARTESIAN_POINT ( 'NONE',  ( -145.0000000000000568, -12.50000000000001066, 15.00000000000001243 ) ) ;
#32793=EDGE_CURVE ( 'NONE', #26941, #23024, #3804, .T. ) ;
#32807=EDGE_LOOP ( 'NONE', ( #30266, #2104, #33951, #5139, #14874, #33148, #24873, #28451, #24167, #16241, #5473 ) ) ;
#32816=DIRECTION ( 'NONE',  ( 0.000000000000000000, -0.000000000000000000, -1.000000000000000000 ) ) ;
#32836=ADVANCED_FACE ( 'NONE', ( #1497 ), #7165, .T. ) ;
#32850=DIRECTION ( 'NONE',  ( 0.000000000000000000, 0.7071067811865489050, 0.7071067811865462405 ) ) ;
#32872=ORIENTED_EDGE ( 'NONE', *, *, #26520, .T. ) ;
#32879=LINE ( 'NONE', #30575, #12826 ) ;
#32882=CIRCLE ( 'NONE', #14159, 12.00000000000001066 ) ;
#32933=SHAPE_DEFINITION_REPRESENTATION ( #33071, #34141 ) ;
#32954=CARTESIAN_POINT ( 'NONE',  ( 145.0000000000000568, -88.29863524074325198, -74.12844257252345415 ) ) ;
#32975=EDGE_CURVE ( 'NONE', #4511, #20828, #21055, .T. ) ;
#33071=PRODUCT_DEFINITION_SHAPE ( 'NONE', 'NONE',  #22952 ) ;
#33095=EDGE_CURVE ( 'NONE', #14920, #10924, #21937, .T. ) ;
#33098=CARTESIAN_POINT ( 'NONE',  ( 145.0000000000000568, -78.33668825982573480, -65.00000000000000000 ) ) ;
#33111=LINE ( 'NONE', #28129, #23776 ) ;
#33148=ORIENTED_EDGE ( 'NONE', *, *, #8386, .T. ) ;
#33187=ADVANCED_FACE ( 'NONE', ( #23507 ), #14819, .F. ) ;
#33215=CARTESIAN_POINT ( 'NONE',  ( -143.0000000000000568, -90.29102463692674974, -73.95413108702814498 ) ) ;
#33269=ORIENTED_EDGE ( 'NONE', *, *, #32793, .T. ) ;
#33282=DIRECTION ( 'NONE',  ( 0.000000000000000000, 1.000000000000000000, 0.000000000000000000 ) ) ;
#33319=CARTESIAN_POINT ( 'NONE',  ( -143.0000000000000568, -175.8248315648716016, -46.05325008164006562 ) ) ;
#33323=LINE ( 'NONE', #9110, #19107 ) ;
#33340=ADVANCED_FACE ( 'NONE', ( #16704 ), #5808, .F. ) ;
#33373=AXIS2_PLACEMENT_3D ( 'NONE', #11169, #27700, #13834 ) ;
#33429=EDGE_CURVE ( 'NONE', #27638, #23842, #30205, .T. ) ;
#33449=ORIENTED_EDGE ( 'NONE', *, *, #2386, .T. ) ;
#33462=ORIENTED_EDGE ( 'NONE', *, *, #18904, .F. ) ;
#33480=DIRECTION ( 'NONE',  ( 0.000000000000000000, 0.000000000000000000, -1.000000000000000000 ) ) ;
#33526=CARTESIAN_POINT ( 'NONE',  ( 145.0000000000000568, 87.50000000000000000, 65.00000000000000000 ) ) ;
#33539=FACE_BOUND ( 'NONE', #7160, .T. ) ;
#33554=CARTESIAN_POINT ( 'NONE',  ( -145.0000000000000568, -78.33668825982573480, -65.00000000000000000 ) ) ;
#33595=CARTESIAN_POINT ( 'NONE',  ( -143.0000000000000568, -78.33668825982579165, -75.00000000000001421 ) ) ;
#33698=DIRECTION ( 'NONE',  ( -1.000000000000000000, 0.000000000000000000, 0.000000000000000000 ) ) ;
#33718=DIRECTION ( 'NONE',  ( 1.000000000000000000, 0.000000000000000000, 0.000000000000000000 ) ) ;
#33735=CYLINDRICAL_SURFACE ( 'NONE', #34417, 12.00000000000001066 ) ;
#33778=CARTESIAN_POINT ( 'NONE',  ( -145.0000000000000568, 87.50000000000000000, 65.00000000000000000 ) ) ;
#33951=ORIENTED_EDGE ( 'NONE', *, *, #6555, .T. ) ;
#33952=DIRECTION ( 'NONE',  ( 0.000000000000000000, 0.000000000000000000, 1.000000000000000000 ) ) ;
#33954=PLANE ( 'NONE',  #31737 ) ;
#33962=LINE ( 'NONE', #31288, #4612 ) ;
#34098=LINE ( 'NONE', #29107, #1828 ) ;
#34134=CIRCLE ( 'NONE', #30221, 11.99999999999999645 ) ;
#34141=SHAPE_REPRESENTATION ( 'top shell', ( #28566 ), #5242 ) ;
#34164=ORIENTED_EDGE ( 'NONE', *, *, #4973, .F. ) ;
#34171=ORIENTED_EDGE ( 'NONE', *, *, #6897, .T. ) ;
#34177=LINE ( 'NONE', #4440, #1129 ) ;
#34179=ORIENTED_EDGE ( 'NONE', *, *, #16410, .F. ) ;
#34221=EDGE_CURVE ( 'NONE', #3001, #10822, #32563, .T. ) ;
#34249=VECTOR ( 'NONE', #26227, 1000.000000000000227 ) ;
#34290=VERTEX_POINT ( 'NONE', #31188 ) ;
#34306=FACE_OUTER_BOUND ( 'NONE', #3329, .T. ) ;
#34315=PLANE ( 'NONE',  #28208 ) ;
#34366=CARTESIAN_POINT ( 'NONE',  ( -145.0000000000000568, -177.8172209610550851, -45.87893859614474223 ) ) ;
#34385=ORIENTED_EDGE ( 'NONE', *, *, #10272, .T. ) ;
#34417=AXIS2_PLACEMENT_3D ( 'NONE', #30719, #11871, #25186 ) ;
#34424=ORIENTED_EDGE ( 'NONE', *, *, #2074, .T. ) ;
#34438=CARTESIAN_POINT ( 'NONE',  ( 143.0000000000000568, -99.56883598056833762, -180.0000000000000000 ) ) ;
#34478=DIRECTION ( 'NONE',  ( 0.000000000000000000, -3.017235169886638201E-16, 1.000000000000000000 ) ) ;
#34484=DIRECTION ( 'NONE',  ( 0.000000000000000000, -0.08715574274766170471, -0.9961946980917453232 ) ) ;
#34495=CARTESIAN_POINT ( 'NONE',  ( 143.0000000000000568, 85.49999999999998579, -63.00000000000000000 ) ) ;
#34499=CARTESIAN_POINT ( 'NONE',  ( 145.0000000000000568, -87.50000000000000000, 65.00000000000000000 ) ) ;
#34524=EDGE_CURVE ( 'NONE', #10781, #27819, #14437, .T. ) ;
#34536=VECTOR ( 'NONE', #4350, 1000.000000000000000 ) ;
#34616=ORIENTED_EDGE ( 'NONE', *, *, #381, .F. ) ;
#34629=DIRECTION ( 'NONE',  ( -1.000000000000000000, 0.000000000000000000, -0.000000000000000000 ) ) ;
#34700=CARTESIAN_POINT ( 'NONE',  ( -145.0000000000000568, -177.8172209610550851, -45.87893859614474223 ) ) ;
#34715=DIRECTION ( 'NONE',  ( -1.000000000000000000, -0.000000000000000000, -0.000000000000000000 ) ) ;
#34770=DIRECTION ( 'NONE',  ( 0.000000000000000000, 0.000000000000000000, -1.000000000000000000 ) ) ;
#34782=ORIENTED_EDGE ( 'NONE', *, *, #7152, .T. ) ;
#34796=DIRECTION ( 'NONE',  ( -0.000000000000000000, 0.08715574274766170471, 0.9961946980917453232 ) ) ;
#34863=FACE_BOUND ( 'NONE', #12808, .T. ) ;
#34864=VERTEX_POINT ( 'NONE', #6171 ) ;
#34932=EDGE_LOOP ( 'NONE', ( #20045, #20053, #1160, #12934 ) ) ;
#34989=LINE ( 'NONE', #12929, #11756 ) ;
#35046=CARTESIAN_POINT ( 'NONE',  ( -143.0000000000000568, -45.49999999999999289, 63.00000000000000000 ) ) ;
#35262=COLOUR_RGB('Sky Blue',0.24,0.69,0.87);
#35263=FILL_AREA_STYLE_COLOUR('',#35262);
#35264=FILL_AREA_STYLE('',(#35263));
#35265=SURFACE_STYLE_FILL_AREA(#35264);
#35266=SURFACE_SIDE_STYLE('',(#35265));
#35267=SURFACE_STYLE_USAGE(.BOTH.,#35266);
#35268=PRESENTATION_STYLE_ASSIGNMENT((#35267));
ENDSEC;
END-ISO-10303-21;
